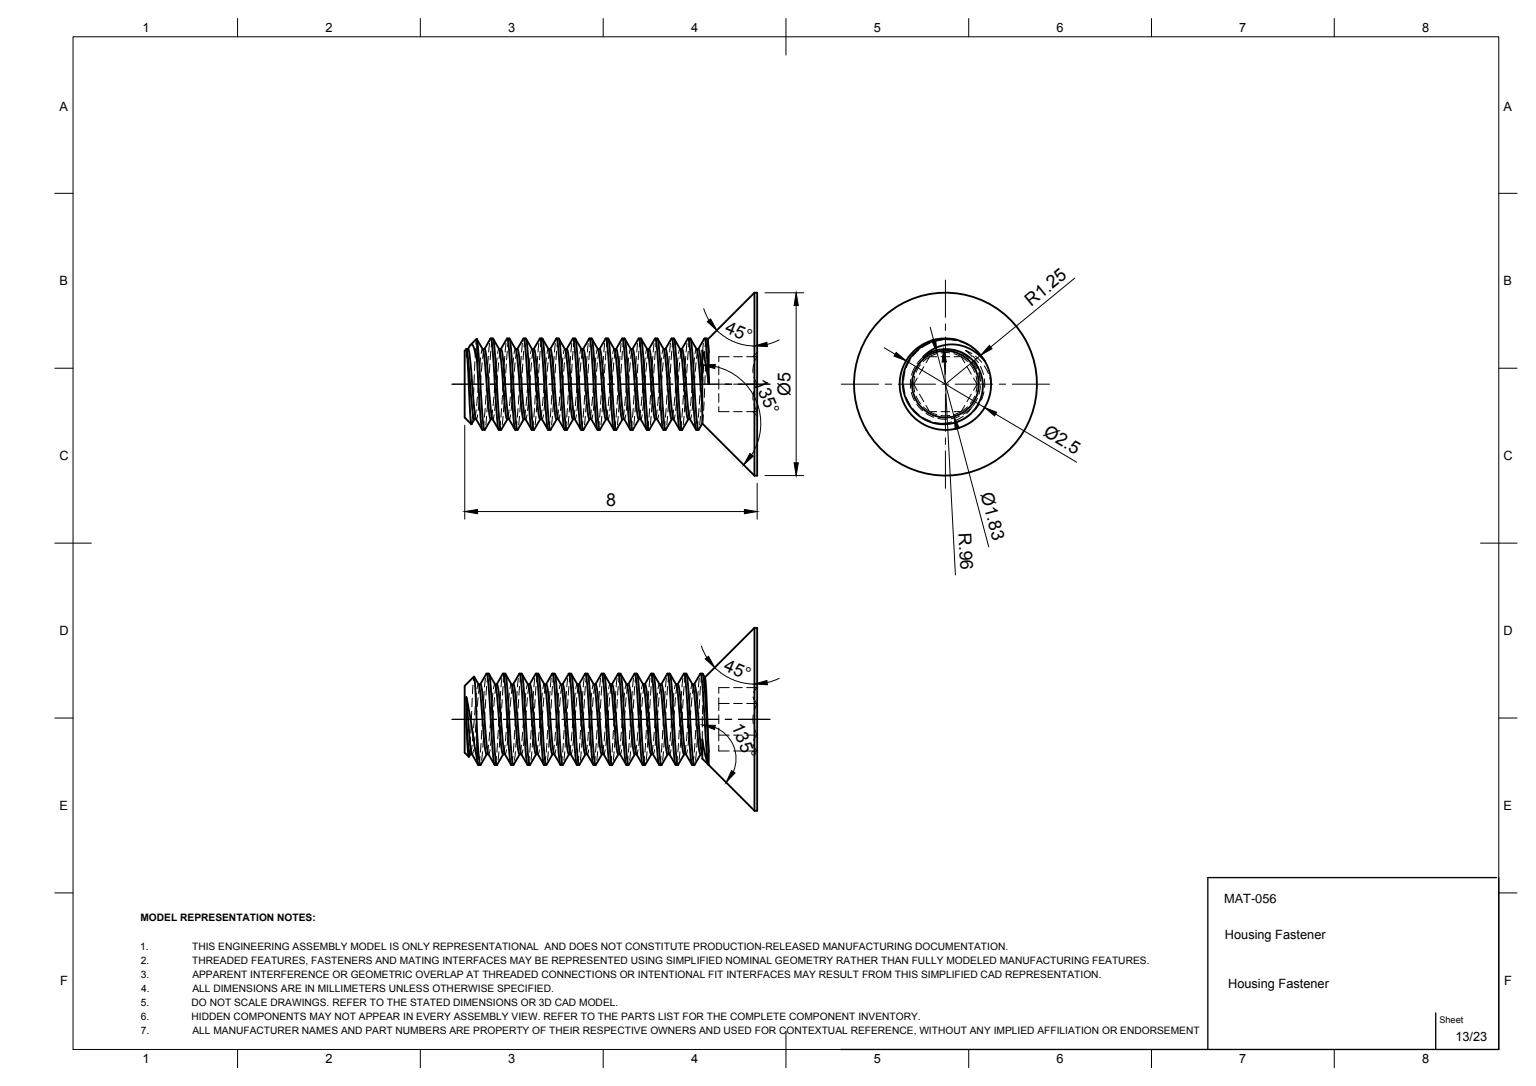
ISO-10303-21;
HEADER;
/* Generated by software containing ST-Developer
 * from STEP Tools, Inc. (www.steptools.com) 
 */

FILE_DESCRIPTION(
/* description */ (''),
/* implementation_level */ '2;1');

FILE_NAME(
/* name */ 'Housing Fastener.step',
/* time_stamp */ '2026-10-28T16:47:13+01:00',
/* author */ (''),
/* organization */ (''),
/* preprocessor_version */ 'ST-DEVELOPER v20.2',
/* originating_system */ 'Autodesk Translation Framework v15.17.0.0',
/* authorisation */ '');

FILE_SCHEMA (('AUTOMOTIVE_DESIGN { 1 0 10303 214 3 1 1 }'));
ENDSEC;

DATA;
#10=MECHANICAL_DESIGN_GEOMETRIC_PRESENTATION_REPRESENTATION('',(#4606),#459242);
#2317=(
BOUNDED_SURFACE()
B_SPLINE_SURFACE(1,2,((#370739,#370740,#370741,#370742,#370743,#370744,
#370745,#370746,#370747,#370748,#370749,#370750,#370751,#370752,#370753,
#370754,#370755,#370756,#370757,#370758,#370759,#370760,#370761,#370762,
#370763,#370764,#370765,#370766,#370767,#370768,#370769,#370770,#370771,
#370772,#370773,#370774,#370775,#370776,#370777,#370778,#370779,#370780,
#370781,#370782,#370783,#370784,#370785,#370786,#370787,#370788,#370789,
#370790,#370791,#370792,#370793,#370794,#370795,#370796,#370797,#370798,
#370799,#370800,#370801,#370802,#370803,#370804,#370805,#370806,#370807,
#370808,#370809,#370810,#370811,#370812,#370813,#370814,#370815,#370816,
#370817,#370818,#370819,#370820,#370821,#370822,#370823,#370824,#370825,
#370826,#370827,#370828,#370829,#370830,#370831,#370832,#370833,#370834,
#370835,#370836,#370837,#370838,#370839,#370840,#370841,#370842,#370843,
#370844,#370845,#370846,#370847,#370848,#370849,#370850,#370851,#370852,
#370853,#370854,#370855,#370856,#370857,#370858,#370859,#370860,#370861,
#370862,#370863,#370864,#370865,#370866,#370867,#370868,#370869,#370870,
#370871,#370872,#370873,#370874,#370875,#370876,#370877,#370878,#370879,
#370880,#370881,#370882,#370883,#370884,#370885,#370886,#370887,#370888,
#370889,#370890,#370891,#370892,#370893,#370894,#370895,#370896,#370897,
#370898,#370899,#370900,#370901,#370902,#370903,#370904,#370905,#370906,
#370907,#370908,#370909,#370910,#370911,#370912,#370913,#370914,#370915,
#370916,#370917,#370918,#370919,#370920,#370921,#370922,#370923,#370924,
#370925,#370926,#370927,#370928,#370929,#370930,#370931,#370932,#370933,
#370934,#370935,#370936,#370937,#370938,#370939,#370940,#370941,#370942,
#370943,#370944,#370945,#370946,#370947,#370948,#370949,#370950,#370951,
#370952,#370953,#370954,#370955),(#370956,#370957,#370958,#370959,#370960,
#370961,#370962,#370963,#370964,#370965,#370966,#370967,#370968,#370969,
#370970,#370971,#370972,#370973,#370974,#370975,#370976,#370977,#370978,
#370979,#370980,#370981,#370982,#370983,#370984,#370985,#370986,#370987,
#370988,#370989,#370990,#370991,#370992,#370993,#370994,#370995,#370996,
#370997,#370998,#370999,#371000,#371001,#371002,#371003,#371004,#371005,
#371006,#371007,#371008,#371009,#371010,#371011,#371012,#371013,#371014,
#371015,#371016,#371017,#371018,#371019,#371020,#371021,#371022,#371023,
#371024,#371025,#371026,#371027,#371028,#371029,#371030,#371031,#371032,
#371033,#371034,#371035,#371036,#371037,#371038,#371039,#371040,#371041,
#371042,#371043,#371044,#371045,#371046,#371047,#371048,#371049,#371050,
#371051,#371052,#371053,#371054,#371055,#371056,#371057,#371058,#371059,
#371060,#371061,#371062,#371063,#371064,#371065,#371066,#371067,#371068,
#371069,#371070,#371071,#371072,#371073,#371074,#371075,#371076,#371077,
#371078,#371079,#371080,#371081,#371082,#371083,#371084,#371085,#371086,
#371087,#371088,#371089,#371090,#371091,#371092,#371093,#371094,#371095,
#371096,#371097,#371098,#371099,#371100,#371101,#371102,#371103,#371104,
#371105,#371106,#371107,#371108,#371109,#371110,#371111,#371112,#371113,
#371114,#371115,#371116,#371117,#371118,#371119,#371120,#371121,#371122,
#371123,#371124,#371125,#371126,#371127,#371128,#371129,#371130,#371131,
#371132,#371133,#371134,#371135,#371136,#371137,#371138,#371139,#371140,
#371141,#371142,#371143,#371144,#371145,#371146,#371147,#371148,#371149,
#371150,#371151,#371152,#371153,#371154,#371155,#371156,#371157,#371158,
#371159,#371160,#371161,#371162,#371163,#371164,#371165,#371166,#371167,
#371168,#371169,#371170,#371171,#371172)),.UNSPECIFIED.,.F.,.F.,.F.)
B_SPLINE_SURFACE_WITH_KNOTS((2,2),(3,2,2,2,2,2,2,2,2,2,2,2,2,2,2,2,2,2,
2,2,2,2,2,2,2,2,2,2,2,2,2,2,2,2,2,2,2,2,2,2,2,2,2,2,2,2,2,2,2,2,2,2,2,2,
2,2,2,2,2,2,2,2,2,2,2,2,2,2,2,2,2,2,2,2,2,2,2,2,2,2,2,2,2,2,2,2,2,2,2,2,
2,2,2,2,2,2,2,2,2,2,2,2,2,2,2,2,2,2,3),(-1.08044907090275E-5,1.),(0.,0.00925925925925926,
0.0185185185185185,0.0277777777777778,0.037037037037037,0.0462962962962963,
0.0555555555555556,0.0648148148148148,0.0740740740740741,0.0833333333333333,
0.0925925925925926,0.101851851851852,0.111111111111111,0.12037037037037,
0.12962962962963,0.138888888888889,0.148148148148148,0.157407407407407,
0.166666666666667,0.175925925925926,0.185185185185185,0.194444444444444,
0.203703703703704,0.212962962962963,0.222222222222222,0.231481481481481,
0.240740740740741,0.25,0.259259259259259,0.268518518518519,0.277777777777778,
0.287037037037037,0.296296296296296,0.305555555555556,0.314814814814815,
0.324074074074074,0.333333333333333,0.342592592592593,0.351851851851852,
0.361111111111111,0.37037037037037,0.37962962962963,0.388888888888889,0.398148148148148,
0.407407407407407,0.416666666666667,0.425925925925926,0.435185185185185,
0.444444444444444,0.453703703703704,0.462962962962963,0.472222222222222,
0.481481481481481,0.490740740740741,0.5,0.509259259259259,0.518518518518518,
0.527777777777778,0.537037037037037,0.546296296296296,0.555555555555556,
0.564814814814815,0.574074074074074,0.583333333333333,0.592592592592593,
0.601851851851852,0.611111111111111,0.62037037037037,0.62962962962963,0.638888888888889,
0.648148148148148,0.657407407407407,0.666666666666667,0.675925925925926,
0.685185185185185,0.694444444444444,0.703703703703704,0.712962962962963,
0.722222222222222,0.731481481481482,0.740740740740741,0.75,0.759259259259259,
0.768518518518518,0.777777777777778,0.787037037037037,0.796296296296296,
0.805555555555556,0.814814814814815,0.824074074074074,0.833333333333333,
0.842592592592593,0.851851851851852,0.861111111111111,0.87037037037037,
0.87962962962963,0.888888888888889,0.898148148148148,0.907407407407407,
0.916666666666667,0.925925925925926,0.935185185185185,0.944444444444444,
0.953703703703704,0.962962962962963,0.972222222222222,0.981481481481482,
0.987622467374972,0.997498692048721),.UNSPECIFIED.)
GEOMETRIC_REPRESENTATION_ITEM()
RATIONAL_B_SPLINE_SURFACE(((1.,0.866025403784439,1.,0.866025403784439,1.,
0.866025403784439,1.,0.866025403784439,1.,0.866025403784439,1.,0.866025403784439,
1.,0.866025403784439,1.,0.866025403784439,1.,0.866025403784439,1.,0.866025403784439,
1.,0.866025403784439,1.,0.866025403784439,1.,0.866025403784439,1.,0.866025403784439,
1.,0.866025403784439,1.,0.866025403784439,1.,0.866025403784439,1.,0.866025403784439,
1.,0.866025403784439,1.,0.866025403784439,1.,0.866025403784439,1.,0.866025403784439,
1.,0.866025403784439,1.,0.866025403784439,1.,0.866025403784439,1.,0.866025403784439,
1.,0.866025403784439,1.,0.866025403784439,1.,0.866025403784439,1.,0.866025403784439,
1.,0.866025403784439,1.,0.866025403784439,1.,0.866025403784439,1.,0.866025403784439,
1.,0.866025403784439,1.,0.866025403784439,1.,0.866025403784439,1.,0.866025403784439,
1.,0.866025403784439,1.,0.866025403784439,1.,0.866025403784439,1.,0.866025403784439,
1.,0.866025403784439,1.,0.866025403784439,1.,0.866025403784439,1.,0.866025403784439,
1.,0.866025403784439,1.,0.866025403784439,1.,0.866025403784439,1.,0.866025403784439,
1.,0.866025403784439,1.,0.866025403784439,1.,0.866025403784439,1.,0.866025403784439,
1.,0.866025403784439,1.,0.866025403784439,1.,0.866025403784439,1.,0.866025403784439,
1.,0.866025403784439,1.,0.866025403784439,1.,0.866025403784439,1.,0.866025403784439,
1.,0.866025403784439,1.,0.866025403784439,1.,0.866025403784439,1.,0.866025403784439,
1.,0.866025403784439,1.,0.866025403784439,1.,0.866025403784439,1.,0.866025403784439,
1.,0.866025403784439,1.,0.866025403784439,1.,0.866025403784439,1.,0.866025403784439,
1.,0.866025403784439,1.,0.866025403784439,1.,0.866025403784439,1.,0.866025403784439,
1.,0.866025403784439,1.,0.866025403784439,1.,0.866025403784439,1.,0.866025403784439,
1.,0.866025403784439,1.,0.866025403784439,1.,0.866025403784439,1.,0.866025403784439,
1.,0.866025403784439,1.,0.866025403784439,1.,0.866025403784439,1.,0.866025403784439,
1.,0.866025403784439,1.,0.866025403784439,1.,0.866025403784439,1.,0.866025403784439,
1.,0.866025403784439,1.,0.866025403784439,1.,0.866025403784439,1.,0.866025403784439,
1.,0.866025403784439,1.,0.866025403784439,1.,0.866025403784439,1.,0.866025403784439,
1.,0.866025403784439,1.,0.866025403784439,1.,0.866025403784439,1.,0.866025403784439,
1.,0.911144500611853,0.940151640776859,0.940151640776859,0.940151640776859),
(1.,0.866025403784439,1.,0.866025403784439,1.,0.866025403784439,1.,0.866025403784439,
1.,0.866025403784439,1.,0.866025403784439,1.,0.866025403784439,1.,0.866025403784439,
1.,0.866025403784439,1.,0.866025403784439,1.,0.866025403784439,1.,0.866025403784439,
1.,0.866025403784439,1.,0.866025403784439,1.,0.866025403784439,1.,0.866025403784439,
1.,0.866025403784439,1.,0.866025403784439,1.,0.866025403784439,1.,0.866025403784439,
1.,0.866025403784439,1.,0.866025403784439,1.,0.866025403784439,1.,0.866025403784439,
1.,0.866025403784439,1.,0.866025403784439,1.,0.866025403784439,1.,0.866025403784439,
1.,0.866025403784439,1.,0.866025403784439,1.,0.866025403784439,1.,0.866025403784439,
1.,0.866025403784439,1.,0.866025403784439,1.,0.866025403784439,1.,0.866025403784439,
1.,0.866025403784439,1.,0.866025403784439,1.,0.866025403784439,1.,0.866025403784439,
1.,0.866025403784439,1.,0.866025403784439,1.,0.866025403784439,1.,0.866025403784439,
1.,0.866025403784439,1.,0.866025403784439,1.,0.866025403784439,1.,0.866025403784439,
1.,0.866025403784439,1.,0.866025403784439,1.,0.866025403784439,1.,0.866025403784439,
1.,0.866025403784439,1.,0.866025403784439,1.,0.866025403784439,1.,0.866025403784439,
1.,0.866025403784439,1.,0.866025403784439,1.,0.866025403784439,1.,0.866025403784439,
1.,0.866025403784439,1.,0.866025403784439,1.,0.866025403784439,1.,0.866025403784439,
1.,0.866025403784439,1.,0.866025403784439,1.,0.866025403784439,1.,0.866025403784439,
1.,0.866025403784439,1.,0.866025403784439,1.,0.866025403784439,1.,0.866025403784439,
1.,0.866025403784439,1.,0.866025403784439,1.,0.866025403784439,1.,0.866025403784439,
1.,0.866025403784439,1.,0.866025403784439,1.,0.866025403784439,1.,0.866025403784439,
1.,0.866025403784439,1.,0.866025403784439,1.,0.866025403784439,1.,0.866025403784439,
1.,0.866025403784439,1.,0.866025403784439,1.,0.866025403784439,1.,0.866025403784439,
1.,0.866025403784439,1.,0.866025403784439,1.,0.866025403784439,1.,0.866025403784439,
1.,0.866025403784439,1.,0.866025403784439,1.,0.866025403784439,1.,0.866025403784439,
1.,0.866025403784439,1.,0.866025403784439,1.,0.866025403784439,1.,0.866025403784439,
1.,0.866025403784439,1.,0.866025403784439,1.,0.866025403784439,1.,0.866025403784439,
1.,0.866025403784439,1.,0.866025403784439,1.,0.911144500611853,0.940151640776859,
0.940151640776859,0.940151640776859)))
REPRESENTATION_ITEM('')
SURFACE()
);
#2318=(
BOUNDED_SURFACE()
B_SPLINE_SURFACE(1,2,((#371177,#371178,#371179,#371180,#371181,#371182,
#371183,#371184,#371185,#371186,#371187,#371188,#371189,#371190,#371191,
#371192,#371193,#371194,#371195,#371196,#371197,#371198,#371199,#371200,
#371201,#371202,#371203,#371204,#371205,#371206,#371207,#371208,#371209,
#371210,#371211,#371212,#371213,#371214,#371215,#371216,#371217,#371218,
#371219,#371220,#371221,#371222,#371223,#371224,#371225,#371226,#371227,
#371228,#371229,#371230,#371231,#371232,#371233,#371234,#371235,#371236,
#371237,#371238,#371239,#371240,#371241,#371242,#371243,#371244,#371245,
#371246,#371247,#371248,#371249,#371250,#371251,#371252,#371253,#371254,
#371255,#371256,#371257,#371258,#371259,#371260,#371261,#371262,#371263,
#371264,#371265,#371266,#371267,#371268,#371269,#371270,#371271,#371272,
#371273,#371274,#371275,#371276,#371277,#371278,#371279,#371280,#371281,
#371282,#371283,#371284,#371285,#371286,#371287,#371288,#371289,#371290,
#371291,#371292,#371293,#371294,#371295,#371296,#371297,#371298,#371299,
#371300,#371301,#371302,#371303,#371304,#371305,#371306,#371307,#371308,
#371309,#371310,#371311,#371312,#371313,#371314,#371315,#371316,#371317,
#371318,#371319,#371320,#371321,#371322,#371323,#371324,#371325,#371326,
#371327,#371328,#371329,#371330,#371331,#371332,#371333,#371334,#371335,
#371336,#371337,#371338,#371339,#371340,#371341,#371342,#371343,#371344,
#371345,#371346,#371347,#371348,#371349,#371350,#371351,#371352,#371353,
#371354,#371355,#371356,#371357,#371358,#371359,#371360,#371361,#371362,
#371363,#371364,#371365,#371366,#371367,#371368,#371369,#371370,#371371,
#371372,#371373,#371374,#371375,#371376,#371377,#371378,#371379,#371380,
#371381,#371382,#371383,#371384,#371385,#371386,#371387,#371388,#371389,
#371390,#371391),(#371392,#371393,#371394,#371395,#371396,#371397,#371398,
#371399,#371400,#371401,#371402,#371403,#371404,#371405,#371406,#371407,
#371408,#371409,#371410,#371411,#371412,#371413,#371414,#371415,#371416,
#371417,#371418,#371419,#371420,#371421,#371422,#371423,#371424,#371425,
#371426,#371427,#371428,#371429,#371430,#371431,#371432,#371433,#371434,
#371435,#371436,#371437,#371438,#371439,#371440,#371441,#371442,#371443,
#371444,#371445,#371446,#371447,#371448,#371449,#371450,#371451,#371452,
#371453,#371454,#371455,#371456,#371457,#371458,#371459,#371460,#371461,
#371462,#371463,#371464,#371465,#371466,#371467,#371468,#371469,#371470,
#371471,#371472,#371473,#371474,#371475,#371476,#371477,#371478,#371479,
#371480,#371481,#371482,#371483,#371484,#371485,#371486,#371487,#371488,
#371489,#371490,#371491,#371492,#371493,#371494,#371495,#371496,#371497,
#371498,#371499,#371500,#371501,#371502,#371503,#371504,#371505,#371506,
#371507,#371508,#371509,#371510,#371511,#371512,#371513,#371514,#371515,
#371516,#371517,#371518,#371519,#371520,#371521,#371522,#371523,#371524,
#371525,#371526,#371527,#371528,#371529,#371530,#371531,#371532,#371533,
#371534,#371535,#371536,#371537,#371538,#371539,#371540,#371541,#371542,
#371543,#371544,#371545,#371546,#371547,#371548,#371549,#371550,#371551,
#371552,#371553,#371554,#371555,#371556,#371557,#371558,#371559,#371560,
#371561,#371562,#371563,#371564,#371565,#371566,#371567,#371568,#371569,
#371570,#371571,#371572,#371573,#371574,#371575,#371576,#371577,#371578,
#371579,#371580,#371581,#371582,#371583,#371584,#371585,#371586,#371587,
#371588,#371589,#371590,#371591,#371592,#371593,#371594,#371595,#371596,
#371597,#371598,#371599,#371600,#371601,#371602,#371603,#371604,#371605,
#371606)),.UNSPECIFIED.,.F.,.F.,.F.)
B_SPLINE_SURFACE_WITH_KNOTS((2,2),(3,2,2,2,2,2,2,2,2,2,2,2,2,2,2,2,2,2,
2,2,2,2,2,2,2,2,2,2,2,2,2,2,2,2,2,2,2,2,2,2,2,2,2,2,2,2,2,2,2,2,2,2,2,2,
2,2,2,2,2,2,2,2,2,2,2,2,2,2,2,2,2,2,2,2,2,2,2,2,2,2,2,2,2,2,2,2,2,2,2,2,
2,2,2,2,2,2,2,2,2,2,2,2,2,2,2,2,2,3),(0.,1.),(0.,0.00925925925925926,0.0185185185185185,
0.0277777777777778,0.037037037037037,0.0462962962962963,0.0555555555555556,
0.0648148148148148,0.0740740740740741,0.0833333333333333,0.0925925925925926,
0.101851851851852,0.111111111111111,0.12037037037037,0.12962962962963,0.138888888888889,
0.148148148148148,0.157407407407407,0.166666666666667,0.175925925925926,
0.185185185185185,0.194444444444444,0.203703703703704,0.212962962962963,
0.222222222222222,0.231481481481481,0.240740740740741,0.25,0.259259259259259,
0.268518518518519,0.277777777777778,0.287037037037037,0.296296296296296,
0.305555555555556,0.314814814814815,0.324074074074074,0.333333333333333,
0.342592592592593,0.351851851851852,0.361111111111111,0.37037037037037,
0.37962962962963,0.388888888888889,0.398148148148148,0.407407407407407,
0.416666666666667,0.425925925925926,0.435185185185185,0.444444444444444,
0.453703703703704,0.462962962962963,0.472222222222222,0.481481481481481,
0.490740740740741,0.5,0.509259259259259,0.518518518518518,0.527777777777778,
0.537037037037037,0.546296296296296,0.555555555555556,0.564814814814815,
0.574074074074074,0.583333333333333,0.592592592592593,0.601851851851852,
0.611111111111111,0.62037037037037,0.62962962962963,0.638888888888889,0.648148148148148,
0.657407407407407,0.666666666666667,0.675925925925926,0.685185185185185,
0.694444444444444,0.703703703703704,0.712962962962963,0.722222222222222,
0.731481481481482,0.740740740740741,0.75,0.759259259259259,0.768518518518518,
0.777777777777778,0.787037037037037,0.796296296296296,0.805555555555556,
0.814814814814815,0.824074074074074,0.833333333333333,0.842592592592593,
0.851851851851852,0.861111111111111,0.87037037037037,0.87962962962963,0.888888888888889,
0.898148148148148,0.907407407407407,0.916666666666667,0.925925925925926,
0.935185185185185,0.944444444444444,0.953703703703704,0.962962962962963,
0.972222222222222,0.981481481481482,0.987622586258463),.UNSPECIFIED.)
GEOMETRIC_REPRESENTATION_ITEM()
RATIONAL_B_SPLINE_SURFACE(((1.,0.866025403784439,1.,0.866025403784439,1.,
0.866025403784439,1.,0.866025403784439,1.,0.866025403784439,1.,0.866025403784439,
1.,0.866025403784439,1.,0.866025403784439,1.,0.866025403784439,1.,0.866025403784439,
1.,0.866025403784439,1.,0.866025403784439,1.,0.866025403784439,1.,0.866025403784439,
1.,0.866025403784439,1.,0.866025403784439,1.,0.866025403784439,1.,0.866025403784439,
1.,0.866025403784439,1.,0.866025403784439,1.,0.866025403784439,1.,0.866025403784439,
1.,0.866025403784439,1.,0.866025403784439,1.,0.866025403784439,1.,0.866025403784439,
1.,0.866025403784439,1.,0.866025403784439,1.,0.866025403784439,1.,0.866025403784439,
1.,0.866025403784439,1.,0.866025403784439,1.,0.866025403784439,1.,0.866025403784439,
1.,0.866025403784439,1.,0.866025403784439,1.,0.866025403784439,1.,0.866025403784439,
1.,0.866025403784439,1.,0.866025403784439,1.,0.866025403784439,1.,0.866025403784439,
1.,0.866025403784439,1.,0.866025403784439,1.,0.866025403784439,1.,0.866025403784439,
1.,0.866025403784439,1.,0.866025403784439,1.,0.866025403784439,1.,0.866025403784439,
1.,0.866025403784439,1.,0.866025403784439,1.,0.866025403784439,1.,0.866025403784439,
1.,0.866025403784439,1.,0.866025403784439,1.,0.866025403784439,1.,0.866025403784439,
1.,0.866025403784439,1.,0.866025403784439,1.,0.866025403784439,1.,0.866025403784439,
1.,0.866025403784439,1.,0.866025403784439,1.,0.866025403784439,1.,0.866025403784439,
1.,0.866025403784439,1.,0.866025403784439,1.,0.866025403784439,1.,0.866025403784439,
1.,0.866025403784439,1.,0.866025403784439,1.,0.866025403784439,1.,0.866025403784439,
1.,0.866025403784439,1.,0.866025403784439,1.,0.866025403784439,1.,0.866025403784439,
1.,0.866025403784439,1.,0.866025403784439,1.,0.866025403784439,1.,0.866025403784439,
1.,0.866025403784439,1.,0.866025403784439,1.,0.866025403784439,1.,0.866025403784439,
1.,0.866025403784439,1.,0.866025403784439,1.,0.866025403784439,1.,0.866025403784439,
1.,0.866025403784439,1.,0.866025403784439,1.,0.866025403784439,1.,0.866025403784439,
1.,0.866025403784439,1.,0.866025403784439,1.,0.866025403784439,1.,0.866025403784439,
1.,0.866025403784439,1.,0.866025403784439,1.,0.866025403784439,1.,0.866025403784439,
1.,0.866025403784439,1.,0.866025403784439,1.,0.866025403784439,1.,0.866025403784439,
1.,0.911142780456138,0.940152763920857),(1.,0.866025403784439,1.,0.866025403784439,
1.,0.866025403784439,1.,0.866025403784439,1.,0.866025403784439,1.,0.866025403784439,
1.,0.866025403784439,1.,0.866025403784439,1.,0.866025403784439,1.,0.866025403784439,
1.,0.866025403784439,1.,0.866025403784439,1.,0.866025403784439,1.,0.866025403784439,
1.,0.866025403784439,1.,0.866025403784439,1.,0.866025403784439,1.,0.866025403784439,
1.,0.866025403784439,1.,0.866025403784439,1.,0.866025403784439,1.,0.866025403784439,
1.,0.866025403784439,1.,0.866025403784439,1.,0.866025403784439,1.,0.866025403784439,
1.,0.866025403784439,1.,0.866025403784439,1.,0.866025403784439,1.,0.866025403784439,
1.,0.866025403784439,1.,0.866025403784439,1.,0.866025403784439,1.,0.866025403784439,
1.,0.866025403784439,1.,0.866025403784439,1.,0.866025403784439,1.,0.866025403784439,
1.,0.866025403784439,1.,0.866025403784439,1.,0.866025403784439,1.,0.866025403784439,
1.,0.866025403784439,1.,0.866025403784439,1.,0.866025403784439,1.,0.866025403784439,
1.,0.866025403784439,1.,0.866025403784439,1.,0.866025403784439,1.,0.866025403784439,
1.,0.866025403784439,1.,0.866025403784439,1.,0.866025403784439,1.,0.866025403784439,
1.,0.866025403784439,1.,0.866025403784439,1.,0.866025403784439,1.,0.866025403784439,
1.,0.866025403784439,1.,0.866025403784439,1.,0.866025403784439,1.,0.866025403784439,
1.,0.866025403784439,1.,0.866025403784439,1.,0.866025403784439,1.,0.866025403784439,
1.,0.866025403784439,1.,0.866025403784439,1.,0.866025403784439,1.,0.866025403784439,
1.,0.866025403784439,1.,0.866025403784439,1.,0.866025403784439,1.,0.866025403784439,
1.,0.866025403784439,1.,0.866025403784439,1.,0.866025403784439,1.,0.866025403784439,
1.,0.866025403784439,1.,0.866025403784439,1.,0.866025403784439,1.,0.866025403784439,
1.,0.866025403784439,1.,0.866025403784439,1.,0.866025403784439,1.,0.866025403784439,
1.,0.866025403784439,1.,0.866025403784439,1.,0.866025403784439,1.,0.866025403784439,
1.,0.866025403784439,1.,0.866025403784439,1.,0.866025403784439,1.,0.866025403784439,
1.,0.866025403784439,1.,0.866025403784439,1.,0.866025403784439,1.,0.866025403784439,
1.,0.866025403784439,1.,0.866025403784439,1.,0.866025403784439,1.,0.866025403784439,
1.,0.866025403784439,1.,0.866025403784439,1.,0.866025403784439,1.,0.866025403784439,
1.,0.911142780456138,0.940152763920857)))
REPRESENTATION_ITEM('')
SURFACE()
);
#4224=(
BOUNDED_CURVE()
B_SPLINE_CURVE(2,(#368993,#368994,#368995,#368996,#368997,#368998,#368999),
 .UNSPECIFIED.,.F.,.F.)
B_SPLINE_CURVE_WITH_KNOTS((3,2,2,3),(0.815651079918082,0.825026379687255,
0.834401679456429,0.840557475565081),.UNSPECIFIED.)
CURVE()
GEOMETRIC_REPRESENTATION_ITEM()
RATIONAL_B_SPLINE_CURVE((1.,0.866025403784439,1.,0.866025403784439,1.,0.912032647664899,
0.939583539764693))
REPRESENTATION_ITEM('')
);
#4225=(
BOUNDED_CURVE()
B_SPLINE_CURVE(2,(#369002,#369003,#369004,#369005,#369006),
 .UNSPECIFIED.,.F.,.F.)
B_SPLINE_CURVE_WITH_KNOTS((3,2,3),(0.815651208026079,0.825026509267758,
0.833532478045858),.UNSPECIFIED.)
CURVE()
GEOMETRIC_REPRESENTATION_ITEM()
RATIONAL_B_SPLINE_CURVE((1.,0.866025403784439,1.,0.878448307623234,0.977458040128596))
REPRESENTATION_ITEM('')
);
#4226=(
BOUNDED_CURVE()
B_SPLINE_CURVE(2,(#369011,#369012,#369013,#369014,#369015,#369016,#369017,
#369018,#369019,#369020,#369021,#369022,#369023),.UNSPECIFIED.,.F.,.F.)
B_SPLINE_CURVE_WITH_KNOTS((3,2,2,2,2,2,3),(0.759399281303043,0.768774581072216,
0.778149880841389,0.787525180610563,0.796900480379736,0.806275780148909,
0.815651079918082),.UNSPECIFIED.)
CURVE()
GEOMETRIC_REPRESENTATION_ITEM()
RATIONAL_B_SPLINE_CURVE((1.,0.866025403784439,1.,0.866025403784439,1.,0.866025403784439,
1.,0.866025403784439,1.,0.866025403784439,1.,0.866025403784439,1.))
REPRESENTATION_ITEM('')
);
#4227=(
BOUNDED_CURVE()
B_SPLINE_CURVE(2,(#369024,#369025,#369026,#369027,#369028,#369029,#369030,
#369031,#369032,#369033,#369034,#369035,#369036),.UNSPECIFIED.,.F.,.F.)
B_SPLINE_CURVE_WITH_KNOTS((3,2,2,2,2,2,3),(0.759399400576005,0.768774701817684,
0.778150003059363,0.787525304301042,0.796900605542721,0.8062759067844,0.815651208026079),
 .UNSPECIFIED.)
CURVE()
GEOMETRIC_REPRESENTATION_ITEM()
RATIONAL_B_SPLINE_CURVE((1.,0.866025403784439,1.,0.866025403784439,1.,0.866025403784439,
1.,0.866025403784439,1.,0.866025403784439,1.,0.866025403784439,1.))
REPRESENTATION_ITEM('')
);
#4228=(
BOUNDED_CURVE()
B_SPLINE_CURVE(2,(#369041,#369042,#369043,#369044,#369045,#369046,#369047,
#369048,#369049,#369050,#369051,#369052,#369053),.UNSPECIFIED.,.F.,.F.)
B_SPLINE_CURVE_WITH_KNOTS((3,2,2,2,2,2,3),(0.703147482688004,0.712522782457177,
0.72189808222635,0.731273381995523,0.740648681764697,0.75002398153387,0.759399281303043),
 .UNSPECIFIED.)
CURVE()
GEOMETRIC_REPRESENTATION_ITEM()
RATIONAL_B_SPLINE_CURVE((1.,0.866025403784439,1.,0.866025403784439,1.,0.866025403784439,
1.,0.866025403784439,1.,0.866025403784439,1.,0.866025403784439,1.))
REPRESENTATION_ITEM('')
);
#4229=(
BOUNDED_CURVE()
B_SPLINE_CURVE(2,(#369054,#369055,#369056,#369057,#369058,#369059,#369060,
#369061,#369062,#369063,#369064,#369065,#369066),.UNSPECIFIED.,.F.,.F.)
B_SPLINE_CURVE_WITH_KNOTS((3,2,2,2,2,2,3),(0.70314759312593,0.712522894367609,
0.721898195609288,0.731273496850967,0.740648798092646,0.750024099334325,
0.759399400576005),.UNSPECIFIED.)
CURVE()
GEOMETRIC_REPRESENTATION_ITEM()
RATIONAL_B_SPLINE_CURVE((1.,0.866025403784439,1.,0.866025403784439,1.,0.866025403784439,
1.,0.866025403784439,1.,0.866025403784439,1.,0.866025403784439,1.))
REPRESENTATION_ITEM('')
);
#4230=(
BOUNDED_CURVE()
B_SPLINE_CURVE(2,(#369071,#369072,#369073,#369074,#369075,#369076,#369077,
#369078,#369079,#369080,#369081,#369082,#369083),.UNSPECIFIED.,.F.,.F.)
B_SPLINE_CURVE_WITH_KNOTS((3,2,2,2,2,2,3),(0.646895684072964,0.656270983842138,
0.665646283611311,0.675021583380484,0.684396883149657,0.693772182918831,
0.703147482688004),.UNSPECIFIED.)
CURVE()
GEOMETRIC_REPRESENTATION_ITEM()
RATIONAL_B_SPLINE_CURVE((1.,0.866025403784439,1.,0.866025403784439,1.,0.866025403784439,
1.,0.866025403784439,1.,0.866025403784439,1.,0.866025403784439,1.))
REPRESENTATION_ITEM('')
);
#4231=(
BOUNDED_CURVE()
B_SPLINE_CURVE(2,(#369084,#369085,#369086,#369087,#369088,#369089,#369090,
#369091,#369092,#369093,#369094,#369095,#369096),.UNSPECIFIED.,.F.,.F.)
B_SPLINE_CURVE_WITH_KNOTS((3,2,2,2,2,2,3),(0.646895785675856,0.656271086917535,
0.665646388159214,0.675021689400893,0.684396990642572,0.693772291884251,
0.70314759312593),.UNSPECIFIED.)
CURVE()
GEOMETRIC_REPRESENTATION_ITEM()
RATIONAL_B_SPLINE_CURVE((1.,0.866025403784439,1.,0.866025403784439,1.,0.866025403784439,
1.,0.866025403784439,1.,0.866025403784439,1.,0.866025403784439,1.))
REPRESENTATION_ITEM('')
);
#4232=(
BOUNDED_CURVE()
B_SPLINE_CURVE(2,(#369101,#369102,#369103,#369104,#369105,#369106,#369107,
#369108,#369109,#369110,#369111,#369112,#369113),.UNSPECIFIED.,.F.,.F.)
B_SPLINE_CURVE_WITH_KNOTS((3,2,2,2,2,2,3),(0.590643885457925,0.600019185227099,
0.609394484996272,0.618769784765445,0.628145084534618,0.637520384303791,
0.646895684072964),.UNSPECIFIED.)
CURVE()
GEOMETRIC_REPRESENTATION_ITEM()
RATIONAL_B_SPLINE_CURVE((1.,0.866025403784439,1.,0.866025403784439,1.,0.866025403784439,
1.,0.866025403784439,1.,0.866025403784439,1.,0.866025403784439,1.))
REPRESENTATION_ITEM('')
);
#4233=(
BOUNDED_CURVE()
B_SPLINE_CURVE(2,(#369114,#369115,#369116,#369117,#369118,#369119,#369120,
#369121,#369122,#369123,#369124,#369125,#369126),.UNSPECIFIED.,.F.,.F.)
B_SPLINE_CURVE_WITH_KNOTS((3,2,2,2,2,2,3),(0.590643978225781,0.60001927946746,
0.60939458070914,0.618769881950819,0.628145183192497,0.637520484434177,
0.646895785675856),.UNSPECIFIED.)
CURVE()
GEOMETRIC_REPRESENTATION_ITEM()
RATIONAL_B_SPLINE_CURVE((1.,0.866025403784439,1.,0.866025403784439,1.,0.866025403784439,
1.,0.866025403784439,1.,0.866025403784439,1.,0.866025403784439,1.))
REPRESENTATION_ITEM('')
);
#4234=(
BOUNDED_CURVE()
B_SPLINE_CURVE(2,(#369131,#369132,#369133,#369134,#369135,#369136,#369137,
#369138,#369139,#369140,#369141,#369142,#369143),.UNSPECIFIED.,.F.,.F.)
B_SPLINE_CURVE_WITH_KNOTS((3,2,2,2,2,2,3),(0.534392086842886,0.543767386612059,
0.553142686381232,0.562517986150406,0.571893285919579,0.581268585688752,
0.590643885457925),.UNSPECIFIED.)
CURVE()
GEOMETRIC_REPRESENTATION_ITEM()
RATIONAL_B_SPLINE_CURVE((1.,0.866025403784439,1.,0.866025403784439,1.,0.866025403784439,
1.,0.866025403784439,1.,0.866025403784439,1.,0.866025403784439,1.))
REPRESENTATION_ITEM('')
);
#4235=(
BOUNDED_CURVE()
B_SPLINE_CURVE(2,(#369144,#369145,#369146,#369147,#369148,#369149,#369150,
#369151,#369152,#369153,#369154,#369155,#369156),.UNSPECIFIED.,.F.,.F.)
B_SPLINE_CURVE_WITH_KNOTS((3,2,2,2,2,2,3),(0.534392170775707,0.543767472017386,
0.553142773259065,0.562518074500744,0.571893375742423,0.581268676984102,
0.590643978225781),.UNSPECIFIED.)
CURVE()
GEOMETRIC_REPRESENTATION_ITEM()
RATIONAL_B_SPLINE_CURVE((1.,0.866025403784439,1.,0.866025403784439,1.,0.866025403784439,
1.,0.866025403784439,1.,0.866025403784439,1.,0.866025403784439,1.))
REPRESENTATION_ITEM('')
);
#4236=(
BOUNDED_CURVE()
B_SPLINE_CURVE(2,(#369161,#369162,#369163,#369164,#369165,#369166,#369167,
#369168,#369169,#369170,#369171,#369172,#369173),.UNSPECIFIED.,.F.,.F.)
B_SPLINE_CURVE_WITH_KNOTS((3,2,2,2,2,2,3),(0.478140288227847,0.48751558799702,
0.496890887766193,0.506266187535366,0.51564148730454,0.525016787073713,
0.534392086842886),.UNSPECIFIED.)
CURVE()
GEOMETRIC_REPRESENTATION_ITEM()
RATIONAL_B_SPLINE_CURVE((1.,0.866025403784439,1.,0.866025403784439,1.,0.866025403784439,
1.,0.866025403784439,1.,0.866025403784439,1.,0.866025403784439,1.))
REPRESENTATION_ITEM('')
);
#4237=(
BOUNDED_CURVE()
B_SPLINE_CURVE(2,(#369174,#369175,#369176,#369177,#369178,#369179,#369180,
#369181,#369182,#369183,#369184,#369185,#369186),.UNSPECIFIED.,.F.,.F.)
B_SPLINE_CURVE_WITH_KNOTS((3,2,2,2,2,2,3),(0.478140363325633,0.487515664567311,
0.496890965808991,0.50626626705067,0.515641568292349,0.525016869534028,
0.534392170775707),.UNSPECIFIED.)
CURVE()
GEOMETRIC_REPRESENTATION_ITEM()
RATIONAL_B_SPLINE_CURVE((1.,0.866025403784439,1.,0.866025403784439,1.,0.866025403784439,
1.,0.866025403784439,1.,0.866025403784439,1.,0.866025403784439,1.))
REPRESENTATION_ITEM('')
);
#4238=(
BOUNDED_CURVE()
B_SPLINE_CURVE(2,(#369191,#369192,#369193,#369194,#369195,#369196,#369197,
#369198,#369199,#369200,#369201,#369202,#369203),.UNSPECIFIED.,.F.,.F.)
B_SPLINE_CURVE_WITH_KNOTS((3,2,2,2,2,2,3),(0.421888489612808,0.431263789381981,
0.440639089151154,0.450014388920327,0.4593896886895,0.468764988458674,0.478140288227847),
 .UNSPECIFIED.)
CURVE()
GEOMETRIC_REPRESENTATION_ITEM()
RATIONAL_B_SPLINE_CURVE((1.,0.866025403784439,1.,0.866025403784439,1.,0.866025403784439,
1.,0.866025403784439,1.,0.866025403784439,1.,0.866025403784439,1.))
REPRESENTATION_ITEM('')
);
#4239=(
BOUNDED_CURVE()
B_SPLINE_CURVE(2,(#369204,#369205,#369206,#369207,#369208,#369209,#369210,
#369211,#369212,#369213,#369214,#369215,#369216),.UNSPECIFIED.,.F.,.F.)
B_SPLINE_CURVE_WITH_KNOTS((3,2,2,2,2,2,3),(0.421888555875558,0.431263857117237,
0.440639158358916,0.450014459600595,0.459389760842274,0.468765062083953,
0.478140363325633),.UNSPECIFIED.)
CURVE()
GEOMETRIC_REPRESENTATION_ITEM()
RATIONAL_B_SPLINE_CURVE((1.,0.866025403784439,1.,0.866025403784439,1.,0.866025403784439,
1.,0.866025403784439,1.,0.866025403784439,1.,0.866025403784439,1.))
REPRESENTATION_ITEM('')
);
#4240=(
BOUNDED_CURVE()
B_SPLINE_CURVE(2,(#369221,#369222,#369223,#369224,#369225,#369226,#369227,
#369228,#369229,#369230,#369231,#369232,#369233),.UNSPECIFIED.,.F.,.F.)
B_SPLINE_CURVE_WITH_KNOTS((3,2,2,2,2,2,3),(0.365636690997768,0.375011990766941,
0.384387290536115,0.393762590305288,0.403137890074461,0.412513189843634,
0.421888489612808),.UNSPECIFIED.)
CURVE()
GEOMETRIC_REPRESENTATION_ITEM()
RATIONAL_B_SPLINE_CURVE((1.,0.866025403784439,1.,0.866025403784439,1.,0.866025403784439,
1.,0.866025403784439,1.,0.866025403784439,1.,0.866025403784439,1.))
REPRESENTATION_ITEM('')
);
#4241=(
BOUNDED_CURVE()
B_SPLINE_CURVE(2,(#369234,#369235,#369236,#369237,#369238,#369239,#369240,
#369241,#369242,#369243,#369244,#369245,#369246),.UNSPECIFIED.,.F.,.F.)
B_SPLINE_CURVE_WITH_KNOTS((3,2,2,2,2,2,3),(0.365636748425484,0.375012049667163,
0.384387350908842,0.393762652150521,0.4031379533922,0.412513254633879,0.421888555875558),
 .UNSPECIFIED.)
CURVE()
GEOMETRIC_REPRESENTATION_ITEM()
RATIONAL_B_SPLINE_CURVE((1.,0.866025403784439,1.,0.866025403784439,1.,0.866025403784439,
1.,0.866025403784439,1.,0.866025403784439,1.,0.866025403784439,1.))
REPRESENTATION_ITEM('')
);
#4242=(
BOUNDED_CURVE()
B_SPLINE_CURVE(2,(#369251,#369252,#369253,#369254,#369255,#369256,#369257,
#369258,#369259,#369260,#369261,#369262,#369263),.UNSPECIFIED.,.F.,.F.)
B_SPLINE_CURVE_WITH_KNOTS((3,2,2,2,2,2,3),(0.309384892382729,0.318760192151902,
0.328135491921075,0.337510791690249,0.346886091459422,0.356261391228595,
0.365636690997768),.UNSPECIFIED.)
CURVE()
GEOMETRIC_REPRESENTATION_ITEM()
RATIONAL_B_SPLINE_CURVE((1.,0.866025403784439,1.,0.866025403784439,1.,0.866025403784439,
1.,0.866025403784439,1.,0.866025403784439,1.,0.866025403784439,1.))
REPRESENTATION_ITEM('')
);
#4243=(
BOUNDED_CURVE()
B_SPLINE_CURVE(2,(#369264,#369265,#369266,#369267,#369268,#369269,#369270,
#369271,#369272,#369273,#369274,#369275,#369276),.UNSPECIFIED.,.F.,.F.)
B_SPLINE_CURVE_WITH_KNOTS((3,2,2,2,2,2,3),(0.309384940975409,0.318760242217088,
0.328135543458767,0.337510844700446,0.346886145942126,0.356261447183805,
0.365636748425484),.UNSPECIFIED.)
CURVE()
GEOMETRIC_REPRESENTATION_ITEM()
RATIONAL_B_SPLINE_CURVE((1.,0.866025403784439,1.,0.866025403784439,1.,0.866025403784439,
1.,0.866025403784439,1.,0.866025403784439,1.,0.866025403784439,1.))
REPRESENTATION_ITEM('')
);
#4244=(
BOUNDED_CURVE()
B_SPLINE_CURVE(2,(#369281,#369282,#369283,#369284,#369285,#369286,#369287,
#369288,#369289,#369290,#369291,#369292,#369293),.UNSPECIFIED.,.F.,.F.)
B_SPLINE_CURVE_WITH_KNOTS((3,2,2,2,2,2,3),(0.25313309376769,0.262508393536863,
0.271883693306036,0.28125899307521,0.290634292844383,0.300009592613556,
0.309384892382729),.UNSPECIFIED.)
CURVE()
GEOMETRIC_REPRESENTATION_ITEM()
RATIONAL_B_SPLINE_CURVE((1.,0.866025403784439,1.,0.866025403784439,1.,0.866025403784439,
1.,0.866025403784439,1.,0.866025403784439,1.,0.866025403784439,1.))
REPRESENTATION_ITEM('')
);
#4245=(
BOUNDED_CURVE()
B_SPLINE_CURVE(2,(#369294,#369295,#369296,#369297,#369298,#369299,#369300,
#369301,#369302,#369303,#369304,#369305,#369306),.UNSPECIFIED.,.F.,.F.)
B_SPLINE_CURVE_WITH_KNOTS((3,2,2,2,2,2,3),(0.253133133525335,0.262508434767014,
0.271883736008693,0.281259037250372,0.290634338492051,0.30000963973373,
0.309384940975409),.UNSPECIFIED.)
CURVE()
GEOMETRIC_REPRESENTATION_ITEM()
RATIONAL_B_SPLINE_CURVE((1.,0.866025403784439,1.,0.866025403784439,1.,0.866025403784439,
1.,0.866025403784439,1.,0.866025403784439,1.,0.866025403784439,1.))
REPRESENTATION_ITEM('')
);
#4246=(
BOUNDED_CURVE()
B_SPLINE_CURVE(2,(#369311,#369312,#369313,#369314,#369315,#369316,#369317,
#369318,#369319,#369320,#369321,#369322,#369323),.UNSPECIFIED.,.F.,.F.)
B_SPLINE_CURVE_WITH_KNOTS((3,2,2,2,2,2,3),(0.196881295152651,0.206256594921824,
0.215631894690997,0.22500719446017,0.234382494229343,0.243757793998517,
0.25313309376769),.UNSPECIFIED.)
CURVE()
GEOMETRIC_REPRESENTATION_ITEM()
RATIONAL_B_SPLINE_CURVE((1.,0.866025403784439,1.,0.866025403784439,1.,0.866025403784439,
1.,0.866025403784439,1.,0.866025403784439,1.,0.866025403784439,1.))
REPRESENTATION_ITEM('')
);
#4247=(
BOUNDED_CURVE()
B_SPLINE_CURVE(2,(#369324,#369325,#369326,#369327,#369328,#369329,#369330,
#369331,#369332,#369333,#369334,#369335,#369336),.UNSPECIFIED.,.F.,.F.)
B_SPLINE_CURVE_WITH_KNOTS((3,2,2,2,2,2,3),(0.19688132607526,0.20625662731694,
0.215631928558619,0.225007229800298,0.234382531041977,0.243757832283656,
0.253133133525335),.UNSPECIFIED.)
CURVE()
GEOMETRIC_REPRESENTATION_ITEM()
RATIONAL_B_SPLINE_CURVE((1.,0.866025403784439,1.,0.866025403784439,1.,0.866025403784439,
1.,0.866025403784439,1.,0.866025403784439,1.,0.866025403784439,1.))
REPRESENTATION_ITEM('')
);
#4248=(
BOUNDED_CURVE()
B_SPLINE_CURVE(2,(#369341,#369342,#369343,#369344,#369345,#369346,#369347,
#369348,#369349,#369350,#369351,#369352,#369353),.UNSPECIFIED.,.F.,.F.)
B_SPLINE_CURVE_WITH_KNOTS((3,2,2,2,2,2,3),(0.140629496537611,0.150004796306785,
0.159380096075958,0.168755395845131,0.178130695614304,0.187505995383477,
0.196881295152651),.UNSPECIFIED.)
CURVE()
GEOMETRIC_REPRESENTATION_ITEM()
RATIONAL_B_SPLINE_CURVE((1.,0.866025403784439,1.,0.866025403784439,1.,0.866025403784439,
1.,0.866025403784439,1.,0.866025403784439,1.,0.866025403784439,1.))
REPRESENTATION_ITEM('')
);
#4249=(
BOUNDED_CURVE()
B_SPLINE_CURVE(2,(#369354,#369355,#369356,#369357,#369358,#369359,#369360,
#369361,#369362,#369363,#369364,#369365,#369366),.UNSPECIFIED.,.F.,.F.)
B_SPLINE_CURVE_WITH_KNOTS((3,2,2,2,2,2,3),(0.140629518625186,0.150004819866865,
0.159380121108544,0.168755422350223,0.178130723591902,0.187506024833581,
0.19688132607526),.UNSPECIFIED.)
CURVE()
GEOMETRIC_REPRESENTATION_ITEM()
RATIONAL_B_SPLINE_CURVE((1.,0.866025403784439,1.,0.866025403784439,1.,0.866025403784439,
1.,0.866025403784439,1.,0.866025403784439,1.,0.866025403784439,1.))
REPRESENTATION_ITEM('')
);
#4250=(
BOUNDED_CURVE()
B_SPLINE_CURVE(2,(#369371,#369372,#369373,#369374,#369375,#369376,#369377,
#369378,#369379,#369380,#369381,#369382,#369383),.UNSPECIFIED.,.F.,.F.)
B_SPLINE_CURVE_WITH_KNOTS((3,2,2,2,2,2,3),(0.0843776979225721,0.0937529976917453,
0.103128297460919,0.112503597230092,0.121878896999265,0.131254196768438,
0.140629496537611),.UNSPECIFIED.)
CURVE()
GEOMETRIC_REPRESENTATION_ITEM()
RATIONAL_B_SPLINE_CURVE((1.,0.866025403784439,1.,0.866025403784439,1.,0.866025403784439,
1.,0.866025403784439,1.,0.866025403784439,1.,0.866025403784439,1.))
REPRESENTATION_ITEM('')
);
#4251=(
BOUNDED_CURVE()
B_SPLINE_CURVE(2,(#369384,#369385,#369386,#369387,#369388,#369389,#369390,
#369391,#369392,#369393,#369394,#369395,#369396),.UNSPECIFIED.,.F.,.F.)
B_SPLINE_CURVE_WITH_KNOTS((3,2,2,2,2,2,3),(0.0843777111751116,0.0937530124167907,
0.10312831365847,0.112503614900149,0.121878916141828,0.131254217383507,
0.140629518625186),.UNSPECIFIED.)
CURVE()
GEOMETRIC_REPRESENTATION_ITEM()
RATIONAL_B_SPLINE_CURVE((1.,0.866025403784439,1.,0.866025403784439,1.,0.866025403784439,
1.,0.866025403784439,1.,0.866025403784439,1.,0.866025403784439,1.))
REPRESENTATION_ITEM('')
);
#4252=(
BOUNDED_CURVE()
B_SPLINE_CURVE(2,(#369403,#369404,#369405,#369406,#369407,#369408,#369409,
#369410,#369411,#369412,#369413,#369414,#369415),.UNSPECIFIED.,.F.,.F.)
B_SPLINE_CURVE_WITH_KNOTS((3,2,2,2,2,2,3),(0.033715912765314,0.0375011990767061,
0.0468764988458793,0.0562517986150525,0.0656270983842257,0.0750023981533989,
0.0843776979225721),.UNSPECIFIED.)
CURVE()
GEOMETRIC_REPRESENTATION_ITEM()
RATIONAL_B_SPLINE_CURVE((0.93549495027976,0.945907627743645,1.,0.866025403784439,
1.,0.866025403784439,1.,0.866025403784439,1.,0.866025403784439,1.,0.866025403784439,
1.))
REPRESENTATION_ITEM('')
);
#4253=(
BOUNDED_CURVE()
B_SPLINE_CURVE(2,(#369416,#369417,#369418,#369419,#369420,#369421,#369422,
#369423,#369424,#369425,#369426,#369427,#369428),.UNSPECIFIED.,.F.,.F.)
B_SPLINE_CURVE_WITH_KNOTS((3,2,2,2,2,2,3),(0.0281259037250372,0.0375012049667163,
0.0468765062083953,0.0562518074500744,0.0656271086917535,0.0750024099334325,
0.0843777111751116),.UNSPECIFIED.)
CURVE()
GEOMETRIC_REPRESENTATION_ITEM()
RATIONAL_B_SPLINE_CURVE((1.,0.866025403784439,1.,0.866025403784439,1.,0.866025403784439,
1.,0.866025403784439,1.,0.866025403784439,1.,0.866025403784439,1.))
REPRESENTATION_ITEM('')
);
#4254=(
BOUNDED_CURVE()
B_SPLINE_CURVE(2,(#370584,#370585,#370586),.UNSPECIFIED.,.F.,.F.)
B_SPLINE_CURVE_WITH_KNOTS((3,3),(0.120361405182823,0.287808339382405),
 .UNSPECIFIED.)
CURVE()
GEOMETRIC_REPRESENTATION_ITEM()
RATIONAL_B_SPLINE_CURVE((1.61880215351743,1.86923171819516,1.61880215351743))
REPRESENTATION_ITEM('')
);
#4255=(
BOUNDED_CURVE()
B_SPLINE_CURVE(2,(#370694,#370695,#370696),.UNSPECIFIED.,.F.,.F.)
B_SPLINE_CURVE_WITH_KNOTS((3,3),(0.120361405182824,0.287808339382406),
 .UNSPECIFIED.)
CURVE()
GEOMETRIC_REPRESENTATION_ITEM()
RATIONAL_B_SPLINE_CURVE((1.61880215351743,1.86923171819516,1.61880215351743))
REPRESENTATION_ITEM('')
);
#4256=(
BOUNDED_CURVE()
B_SPLINE_CURVE(2,(#370698,#370699,#370700),.UNSPECIFIED.,.F.,.F.)
B_SPLINE_CURVE_WITH_KNOTS((3,3),(0.120361405182823,0.287808339382407),
 .UNSPECIFIED.)
CURVE()
GEOMETRIC_REPRESENTATION_ITEM()
RATIONAL_B_SPLINE_CURVE((1.61880215351743,1.86923171819516,1.61880215351743))
REPRESENTATION_ITEM('')
);
#4257=(
BOUNDED_CURVE()
B_SPLINE_CURVE(2,(#370702,#370703,#370704),.UNSPECIFIED.,.F.,.F.)
B_SPLINE_CURVE_WITH_KNOTS((3,3),(0.120361405182823,0.287808339382406),
 .UNSPECIFIED.)
CURVE()
GEOMETRIC_REPRESENTATION_ITEM()
RATIONAL_B_SPLINE_CURVE((1.61880215351743,1.86923171819516,1.61880215351743))
REPRESENTATION_ITEM('')
);
#4258=(
BOUNDED_CURVE()
B_SPLINE_CURVE(2,(#370706,#370707,#370708),.UNSPECIFIED.,.F.,.F.)
B_SPLINE_CURVE_WITH_KNOTS((3,3),(0.120361405182824,0.287808339382405),
 .UNSPECIFIED.)
CURVE()
GEOMETRIC_REPRESENTATION_ITEM()
RATIONAL_B_SPLINE_CURVE((1.61880215351743,1.86923171819515,1.61880215351743))
REPRESENTATION_ITEM('')
);
#4259=(
BOUNDED_CURVE()
B_SPLINE_CURVE(2,(#370710,#370711,#370712),.UNSPECIFIED.,.F.,.F.)
B_SPLINE_CURVE_WITH_KNOTS((3,3),(0.120361405182823,0.287808339382406),
 .UNSPECIFIED.)
CURVE()
GEOMETRIC_REPRESENTATION_ITEM()
RATIONAL_B_SPLINE_CURVE((1.61880215351743,1.86923171819516,1.61880215351743))
REPRESENTATION_ITEM('')
);
#4260=(
BOUNDED_CURVE()
B_SPLINE_CURVE(2,(#371174,#371175,#371176),.UNSPECIFIED.,.F.,.F.)
B_SPLINE_CURVE_WITH_KNOTS((3,3),(0.0266276333531501,0.0281259037250372),
 .UNSPECIFIED.)
CURVE()
GEOMETRIC_REPRESENTATION_ITEM()
RATIONAL_B_SPLINE_CURVE((0.964022189566802,0.978589470042526,1.))
REPRESENTATION_ITEM('')
);
#4418=SHAPE_REPRESENTATION_RELATIONSHIP('SRR','None',#459344,#4439);
#4439=ADVANCED_BREP_SHAPE_REPRESENTATION('',(#4486),#459233);
#4486=MANIFOLD_SOLID_BREP('Body1',#94664);
#4606=STYLED_ITEM('',(#459533),#4486);
#4895=CONICAL_SURFACE('',#99351,1.25000000000001,0.78539816339745);
#4896=CONICAL_SURFACE('',#99356,0.866025403784441,0.78539816339745);
#4897=CONICAL_SURFACE('',#99361,2.5,0.785398163397448);
#4898=CONICAL_SURFACE('',#99371,0.866025403784441,0.78539816339745);
#4899=CONICAL_SURFACE('',#99372,0.866025403784441,0.78539816339745);
#4900=CONICAL_SURFACE('',#99373,0.866025403784441,0.78539816339745);
#4901=CONICAL_SURFACE('',#99374,0.866025403784441,0.78539816339745);
#4902=CONICAL_SURFACE('',#99375,0.866025403784441,0.78539816339745);
#5225=FACE_BOUND('',#14454,.T.);
#5716=PLANE('',#99364);
#5717=PLANE('',#99370);
#5718=PLANE('',#99376);
#5719=PLANE('',#99377);
#5720=PLANE('',#99378);
#5721=PLANE('',#99379);
#5722=PLANE('',#99380);
#5723=PLANE('',#99381);
#5724=PLANE('',#99382);
#5725=PLANE('',#99383);
#8499=FACE_OUTER_BOUND('',#14419,.T.);
#8500=FACE_OUTER_BOUND('',#14420,.T.);
#8501=FACE_OUTER_BOUND('',#14421,.T.);
#8502=FACE_OUTER_BOUND('',#14422,.T.);
#8503=FACE_OUTER_BOUND('',#14423,.T.);
#8504=FACE_OUTER_BOUND('',#14424,.T.);
#8505=FACE_OUTER_BOUND('',#14425,.T.);
#8506=FACE_OUTER_BOUND('',#14426,.T.);
#8507=FACE_OUTER_BOUND('',#14427,.T.);
#8508=FACE_OUTER_BOUND('',#14428,.T.);
#8509=FACE_OUTER_BOUND('',#14429,.T.);
#8510=FACE_OUTER_BOUND('',#14430,.T.);
#8511=FACE_OUTER_BOUND('',#14431,.T.);
#8512=FACE_OUTER_BOUND('',#14432,.T.);
#8513=FACE_OUTER_BOUND('',#14433,.T.);
#8514=FACE_OUTER_BOUND('',#14434,.T.);
#8515=FACE_OUTER_BOUND('',#14435,.T.);
#8516=FACE_OUTER_BOUND('',#14436,.T.);
#8517=FACE_OUTER_BOUND('',#14437,.T.);
#8518=FACE_OUTER_BOUND('',#14438,.T.);
#8519=FACE_OUTER_BOUND('',#14439,.T.);
#8520=FACE_OUTER_BOUND('',#14440,.T.);
#8521=FACE_OUTER_BOUND('',#14441,.T.);
#8522=FACE_OUTER_BOUND('',#14442,.T.);
#8523=FACE_OUTER_BOUND('',#14443,.T.);
#8524=FACE_OUTER_BOUND('',#14444,.T.);
#8525=FACE_OUTER_BOUND('',#14445,.T.);
#8526=FACE_OUTER_BOUND('',#14446,.T.);
#8527=FACE_OUTER_BOUND('',#14447,.T.);
#8528=FACE_OUTER_BOUND('',#14448,.T.);
#8529=FACE_OUTER_BOUND('',#14449,.T.);
#8530=FACE_OUTER_BOUND('',#14450,.T.);
#8531=FACE_OUTER_BOUND('',#14451,.T.);
#8532=FACE_OUTER_BOUND('',#14452,.T.);
#8533=FACE_OUTER_BOUND('',#14453,.T.);
#8534=FACE_OUTER_BOUND('',#14455,.T.);
#8535=FACE_OUTER_BOUND('',#14456,.T.);
#8536=FACE_OUTER_BOUND('',#14457,.T.);
#8537=FACE_OUTER_BOUND('',#14458,.T.);
#8538=FACE_OUTER_BOUND('',#14459,.T.);
#8539=FACE_OUTER_BOUND('',#14460,.T.);
#8540=FACE_OUTER_BOUND('',#14461,.T.);
#8541=FACE_OUTER_BOUND('',#14462,.T.);
#8542=FACE_OUTER_BOUND('',#14463,.T.);
#8543=FACE_OUTER_BOUND('',#14464,.T.);
#8544=FACE_OUTER_BOUND('',#14465,.T.);
#8545=FACE_OUTER_BOUND('',#14466,.T.);
#8546=FACE_OUTER_BOUND('',#14467,.T.);
#8547=FACE_OUTER_BOUND('',#14468,.T.);
#8548=FACE_OUTER_BOUND('',#14469,.T.);
#8549=FACE_OUTER_BOUND('',#14470,.T.);
#8550=FACE_OUTER_BOUND('',#14471,.T.);
#14419=EDGE_LOOP('',(#69656,#69657,#69658,#69659));
#14420=EDGE_LOOP('',(#69660,#69661,#69662,#69663));
#14421=EDGE_LOOP('',(#69664,#69665,#69666,#69667));
#14422=EDGE_LOOP('',(#69668,#69669,#69670,#69671));
#14423=EDGE_LOOP('',(#69672,#69673,#69674,#69675));
#14424=EDGE_LOOP('',(#69676,#69677,#69678,#69679));
#14425=EDGE_LOOP('',(#69680,#69681,#69682,#69683));
#14426=EDGE_LOOP('',(#69684,#69685,#69686,#69687));
#14427=EDGE_LOOP('',(#69688,#69689,#69690,#69691));
#14428=EDGE_LOOP('',(#69692,#69693,#69694,#69695));
#14429=EDGE_LOOP('',(#69696,#69697,#69698,#69699));
#14430=EDGE_LOOP('',(#69700,#69701,#69702,#69703));
#14431=EDGE_LOOP('',(#69704,#69705,#69706,#69707));
#14432=EDGE_LOOP('',(#69708,#69709,#69710,#69711));
#14433=EDGE_LOOP('',(#69712,#69713,#69714,#69715,#69716));
#14434=EDGE_LOOP('',(#69717,#69718,#69719,#69720));
#14435=EDGE_LOOP('',(#69721,#69722,#69723,#69724));
#14436=EDGE_LOOP('',(#69725,#69726,#69727,#69728));
#14437=EDGE_LOOP('',(#69729,#69730,#69731,#69732));
#14438=EDGE_LOOP('',(#69733,#69734,#69735,#69736));
#14439=EDGE_LOOP('',(#69737,#69738,#69739,#69740));
#14440=EDGE_LOOP('',(#69741,#69742,#69743,#69744));
#14441=EDGE_LOOP('',(#69745,#69746,#69747,#69748));
#14442=EDGE_LOOP('',(#69749,#69750,#69751,#69752));
#14443=EDGE_LOOP('',(#69753,#69754,#69755,#69756));
#14444=EDGE_LOOP('',(#69757,#69758,#69759,#69760));
#14445=EDGE_LOOP('',(#69761,#69762,#69763,#69764));
#14446=EDGE_LOOP('',(#69765,#69766,#69767,#69768));
#14447=EDGE_LOOP('',(#69769,#69770,#69771,#69772));
#14448=EDGE_LOOP('',(#69773,#69774,#69775,#69776,#69777,#69778,#69779,#69780,
#69781));
#14449=EDGE_LOOP('',(#69782,#69783,#69784,#69785));
#14450=EDGE_LOOP('',(#69786,#69787));
#14451=EDGE_LOOP('',(#69788,#69789,#69790,#69791));
#14452=EDGE_LOOP('',(#69792,#69793,#69794,#69795,#69796,#69797,#69798,#69799));
#14453=EDGE_LOOP('',(#69800));
#14454=EDGE_LOOP('',(#69801,#69802,#69803,#69804,#69805,#69806));
#14455=EDGE_LOOP('',(#69807,#69808,#69809,#69810,#69811));
#14456=EDGE_LOOP('',(#69812,#69813));
#14457=EDGE_LOOP('',(#69814,#69815));
#14458=EDGE_LOOP('',(#69816,#69817));
#14459=EDGE_LOOP('',(#69818,#69819));
#14460=EDGE_LOOP('',(#69820,#69821));
#14461=EDGE_LOOP('',(#69822,#69823,#69824,#69825,#69826,#69827));
#14462=EDGE_LOOP('',(#69828,#69829,#69830,#69831));
#14463=EDGE_LOOP('',(#69832,#69833,#69834,#69835));
#14464=EDGE_LOOP('',(#69836,#69837,#69838,#69839));
#14465=EDGE_LOOP('',(#69840,#69841,#69842,#69843));
#14466=EDGE_LOOP('',(#69844,#69845,#69846,#69847));
#14467=EDGE_LOOP('',(#69848,#69849,#69850,#69851));
#14468=EDGE_LOOP('',(#69852));
#14469=EDGE_LOOP('',(#69853,#69854,#69855,#69856,#69857,#69858,#69859,#69860,
#69861,#69862,#69863,#69864,#69865,#69866,#69867,#69868,#69869,#69870,#69871,
#69872,#69873,#69874,#69875,#69876,#69877,#69878,#69879,#69880,#69881,#69882,
#69883,#69884,#69885,#69886));
#14470=EDGE_LOOP('',(#69887,#69888,#69889));
#14471=EDGE_LOOP('',(#69890,#69891,#69892,#69893,#69894,#69895,#69896,#69897,
#69898,#69899,#69900,#69901,#69902,#69903,#69904,#69905,#69906,#69907,#69908,
#69909,#69910,#69911,#69912,#69913,#69914,#69915,#69916,#69917,#69918,#69919,
#69920,#69921,#69922,#69923));
#20590=CIRCLE('',#99320,0.957716426222737);
#20591=CIRCLE('',#99335,0.957716426224497);
#20592=CIRCLE('',#99337,1.25000000000001);
#20593=CIRCLE('',#99352,0.957716426224497);
#20594=CIRCLE('',#99353,0.912499999999999);
#20595=CIRCLE('',#99355,1.25000000000001);
#20596=CIRCLE('',#99357,0.866025403784441);
#20597=CIRCLE('',#99359,2.5);
#20598=CIRCLE('',#99360,2.5);
#20599=CIRCLE('',#99362,1.075);
#20600=CIRCLE('',#99363,1.075);
#20601=CIRCLE('',#99365,0.866025403784441);
#20602=CIRCLE('',#99366,0.866025403784441);
#20603=CIRCLE('',#99367,0.866025403784441);
#20604=CIRCLE('',#99368,0.866025403784441);
#20605=CIRCLE('',#99369,0.866025403784441);
#24674=B_SPLINE_CURVE_WITH_KNOTS('',3,(#369434,#369435,#369436,#369437,
#369438,#369439,#369440,#369441,#369442,#369443,#369444,#369445,#369446,
#369447,#369448,#369449),.UNSPECIFIED.,.F.,.F.,(4,2,2,2,2,2,2,4),(-0.297225196933553,
-0.280367832092781,-0.230062986451411,-0.181680660100882,-0.132941021745363,
-0.0832685681768193,-0.0412377906385104,-1.00000019265245E-6),
 .UNSPECIFIED.);
#24675=B_SPLINE_CURVE_WITH_KNOTS('',3,(#369452,#369453,#369454,#369455,
#369456,#369457,#369458,#369459,#369460,#369461,#369462,#369463),
 .UNSPECIFIED.,.F.,.F.,(4,2,2,2,2,4),(-11.0969330641696,-11.0506498768724,
-11.0060400646789,-10.9574795152701,-10.9078210422652,-10.9002432379435),
 .UNSPECIFIED.);
#24676=B_SPLINE_CURVE_WITH_KNOTS('',3,(#369468,#369469,#369470,#369471,
#369472,#369473,#369474,#369475,#369476,#369477,#369478,#369479,#369480,
#369481,#369482,#369483,#369484,#369485,#369486,#369487,#369488,#369489,
#369490,#369491,#369492,#369493,#369494,#369495,#369496,#369497,#369498,
#369499,#369500,#369501,#369502,#369503),.UNSPECIFIED.,.F.,.F.,(4,2,2,2,
2,2,2,2,2,2,2,2,2,2,2,2,2,4),(-1.08629683604889,-1.06212709216772,-1.01217701512861,
-0.964116528793942,-0.914651515668606,-0.865348804113709,-0.817791776405739,
-0.768003359154763,-0.719235136420373,-0.671389710240228,-0.621277273749783,
-0.573069866056996,-0.524011681351026,-0.474536688662335,-0.426872955991605,
-0.377053394668109,-0.328108386382734,-0.297225196933553),.UNSPECIFIED.);
#24677=B_SPLINE_CURVE_WITH_KNOTS('',3,(#369504,#369505,#369506,#369507,
#369508,#369509,#369510,#369511,#369512,#369513,#369514,#369515,#369516,
#369517,#369518,#369519,#369520,#369521,#369522,#369523,#369524,#369525,
#369526,#369527,#369528,#369529,#369530,#369531,#369532,#369533,#369534,
#369535,#369536,#369537,#369538,#369539),.UNSPECIFIED.,.F.,.F.,(4,2,2,2,
2,2,2,2,2,2,2,2,2,2,2,2,2,4),(-10.9002432379435,-10.8604065333801,-10.8113104443889,
-10.761713814826,-10.7138417906742,-10.6640923927412,-10.616045003083,-10.5676123012695,
-10.5179413964518,-10.470506852643,-10.4215353486384,-10.371439901378,-10.3236642057133,
-10.2740225073813,-10.2256879132737,-10.1773476975794,-10.1276391307857,
-10.1132239534235),.UNSPECIFIED.);
#24678=B_SPLINE_CURVE_WITH_KNOTS('',3,(#369544,#369545,#369546,#369547,
#369548,#369549,#369550,#369551,#369552,#369553,#369554,#369555,#369556,
#369557,#369558,#369559,#369560,#369561,#369562,#369563,#369564,#369565,
#369566,#369567,#369568,#369569,#369570,#369571,#369572,#369573,#369574,
#369575,#369576,#369577,#369578,#369579),.UNSPECIFIED.,.F.,.F.,(4,2,2,2,
2,2,2,2,2,2,2,2,2,2,2,2,2,4),(-1.87536861874309,-1.84355584199448,-1.79384949462906,
-1.74600741502996,-1.69621082068226,-1.64716056762169,-1.59957435410145,
-1.5497648282856,-1.5012562446633,-1.45296588180679,-1.40314413691098,-1.35519906350488,
-1.305259866274,-1.25610014245001,-1.20856696990882,-1.15878121320228,-1.11015973495678,
-1.08629683604889),.UNSPECIFIED.);
#24679=B_SPLINE_CURVE_WITH_KNOTS('',3,(#369580,#369581,#369582,#369583,
#369584,#369585,#369586,#369587,#369588,#369589,#369590,#369591,#369592,
#369593,#369594,#369595,#369596,#369597,#369598,#369599,#369600,#369601,
#369602,#369603,#369604,#369605,#369606,#369607,#369608,#369609,#369610,
#369611,#369612,#369613,#369614,#369615),.UNSPECIFIED.,.F.,.F.,(4,2,2,2,
2,2,2,2,2,2,2,2,2,2,2,2,2,4),(-10.1132239534235,-10.0801144057446,-10.0312319726685,
-9.98154103730301,-9.93385667477381,-9.88431791432676,-9.83555841579789,
-9.78730128208498,-9.73712994715777,-9.68943338837994,-9.64061521762979,
-9.59087875638848,-9.54332419146615,-9.49397528474752,-9.44486869631985,
-9.3967780067164,-9.34679000923077,-9.3251899560265),.UNSPECIFIED.);
#24680=B_SPLINE_CURVE_WITH_KNOTS('',3,(#369620,#369621,#369622,#369623,
#369624,#369625,#369626,#369627,#369628,#369629,#369630,#369631,#369632,
#369633,#369634,#369635,#369636,#369637,#369638,#369639,#369640,#369641,
#369642,#369643,#369644,#369645,#369646,#369647,#369648,#369649,#369650,
#369651,#369652,#369653,#369654,#369655),.UNSPECIFIED.,.F.,.F.,(4,2,2,2,
2,2,2,2,2,2,2,2,2,2,2,2,2,4),(-2.66450830210884,-2.62523893706397,-2.57591415214878,
-2.52835492082748,-2.47857795237277,-2.42978650601587,-2.38198894395603,
-2.33185002481024,-2.28361946775828,-2.23466059104454,-2.18515729676512,
-2.1374720120089,-2.08765685324303,-2.03868217100641,-1.99096903863913,
-1.94063103897361,-1.89221929222858,-1.87536861874309),.UNSPECIFIED.);
#24681=B_SPLINE_CURVE_WITH_KNOTS('',3,(#369656,#369657,#369658,#369659,
#369660,#369661,#369662,#369663,#369664,#369665,#369666,#369667,#369668,
#369669,#369670,#369671,#369672,#369673,#369674,#369675,#369676,#369677,
#369678,#369679,#369680,#369681,#369682,#369683,#369684,#369685,#369686,
#369687,#369688,#369689,#369690,#369691),.UNSPECIFIED.,.F.,.F.,(4,2,2,2,
2,2,2,2,2,2,2,2,2,2,2,2,2,4),(-9.3251899560265,-9.29896232620477,-9.25031178750326,
-9.20059733433329,-9.15312351256986,-9.10393801333592,-9.05440164539032,
-9.00644825470644,-8.95661223118013,-8.90857392265958,-8.86005981037984,
-8.81033962393501,-8.76286474277573,-8.71381206706934,-8.66378663798527,
-8.61593806564963,-8.56621891848283,-8.53743262087695),.UNSPECIFIED.);
#24682=B_SPLINE_CURVE_WITH_KNOTS('',3,(#369696,#369697,#369698,#369699,
#369700,#369701,#369702,#369703,#369704,#369705,#369706,#369707,#369708,
#369709,#369710,#369711,#369712,#369713,#369714,#369715,#369716,#369717,
#369718,#369719,#369720,#369721,#369722,#369723,#369724,#369725,#369726,
#369727,#369728,#369729,#369730,#369731),.UNSPECIFIED.,.F.,.F.,(4,2,2,2,
2,2,2,2,2,2,2,2,2,2,2,2,2,4),(-3.45311041785451,-3.40640578800035,-3.35734889527748,
-3.30979687791647,-3.26001136181265,-3.21149516431656,-3.16328629585956,
-3.11345375633878,-3.06550007523919,-3.01569323829511,-2.96651867048036,
-2.91900255270055,-2.86923473474433,-2.8205974011257,-2.77263121805615,
-2.72266205646393,-2.6745852915141,-2.66450830210884),.UNSPECIFIED.);
#24683=B_SPLINE_CURVE_WITH_KNOTS('',3,(#369732,#369733,#369734,#369735,
#369736,#369737,#369738,#369739,#369740,#369741,#369742,#369743,#369744,
#369745,#369746,#369747,#369748,#369749,#369750,#369751,#369752,#369753,
#369754,#369755,#369756,#369757,#369758,#369759,#369760,#369761,#369762,
#369763,#369764,#369765,#369766,#369767),.UNSPECIFIED.,.F.,.F.,(4,2,2,2,
2,2,2,2,2,2,2,2,2,2,2,2,2,4),(-8.53743262087695,-8.51790557886756,-8.4694930188994,
-8.41974122096977,-8.37219191612705,-8.32323738821537,-8.27350131454077,
-8.22574932274126,-8.17613872282825,-8.12742281473662,-8.07909951276689,
-8.0288568753523,-7.98115537034797,-7.9322702522769,-7.8825002114564,-7.83489172319436,
-7.7854767277125,-7.74885616038243),.UNSPECIFIED.);
#24684=B_SPLINE_CURVE_WITH_KNOTS('',3,(#369772,#369773,#369774,#369775,
#369776,#369777,#369778,#369779,#369780,#369781,#369782,#369783,#369784,
#369785,#369786,#369787,#369788,#369789,#369790,#369791,#369792,#369793,
#369794,#369795,#369796,#369797,#369798,#369799,#369800,#369801,#369802,
#369803,#369804,#369805,#369806,#369807,#369808,#369809),.UNSPECIFIED.,
 .F.,.F.,(4,2,2,2,2,2,2,2,2,2,2,2,2,2,2,2,2,2,4),(-4.24192213155039,-4.23809792147632,
-4.18836234856388,-4.13957498951885,-4.09185274799052,-4.04171529566761,
-3.9934886596208,-3.94465978359765,-3.89515592670361,-3.84747283207717,
-3.79769147839944,-3.74871439112587,-3.7010548294868,-3.65071175267311,
-3.60229775019791,-3.55373929331727,-3.50402693278433,-3.45618073503253,
-3.45311041785451),.UNSPECIFIED.);
#24685=B_SPLINE_CURVE_WITH_KNOTS('',3,(#369810,#369811,#369812,#369813,
#369814,#369815,#369816,#369817,#369818,#369819,#369820,#369821,#369822,
#369823,#369824,#369825,#369826,#369827,#369828,#369829,#369830,#369831,
#369832,#369833,#369834,#369835,#369836,#369837,#369838,#369839,#369840,
#369841,#369842,#369843,#369844,#369845),.UNSPECIFIED.,.F.,.F.,(4,2,2,2,
2,2,2,2,2,2,2,2,2,2,2,2,2,4),(-7.74885616038243,-7.73643534531436,-7.68828489874703,
-7.63823245858939,-7.59041958736585,-7.54170890559822,-7.49196769011302,
-7.44445938896145,-7.39521440060387,-7.34576049706096,-7.2977545191574,
-7.24786179061972,-7.19985584140599,-7.15128928192139,-7.10154861462626,
-7.05405787738374,-7.00495329873603,-6.96074678199533),.UNSPECIFIED.);
#24686=B_SPLINE_CURVE_WITH_KNOTS('',3,(#369850,#369851,#369852,#369853,
#369854,#369855,#369856,#369857,#369858,#369859,#369860,#369861,#369862,
#369863,#369864,#369865,#369866,#369867,#369868,#369869,#369870,#369871,
#369872,#369873,#369874,#369875,#369876,#369877,#369878,#369879,#369880,
#369881,#369882,#369883,#369884,#369885),.UNSPECIFIED.,.F.,.F.,(4,2,2,2,
2,2,2,2,2,2,2,2,2,2,2,2,2,4),(-5.02972443161939,-5.0187363541838,-4.96900575987408,
-4.92050955509127,-4.87241366245925,-4.82259855136958,-4.77466360731621,
-4.72502503301001,-4.67586344949185,-4.62839019418675,-4.57867076701161,
-4.53004498522224,-4.48217452916704,-4.43221432415173,-4.38414845254951,
-4.33495397914721,-4.28563488367131,-4.24192213155039),.UNSPECIFIED.);
#24687=B_SPLINE_CURVE_WITH_KNOTS('',3,(#369886,#369887,#369888,#369889,
#369890,#369891,#369892,#369893,#369894,#369895,#369896,#369897,#369898,
#369899,#369900,#369901,#369902,#369903,#369904,#369905,#369906,#369907,
#369908,#369909,#369910,#369911,#369912,#369913,#369914,#369915,#369916,
#369917,#369918,#369919,#369920,#369921,#369922,#369923),.UNSPECIFIED.,
 .F.,.F.,(4,2,2,2,2,2,2,2,2,2,2,2,2,2,2,2,2,2,4),(-6.96074678199533,-6.95502152207767,
-6.90527708144643,-6.85655770199055,-6.80874804770292,-6.75868624361776,
-6.71052715808686,-6.66149720058363,-6.61207258246791,-6.56445611871926,
-6.51468173086547,-6.46578683168715,-6.41808529513843,-6.36783220114316,
-6.31949923703344,-6.27079116033409,-6.2211700228527,-6.17340813772743,
-6.17206263548208),.UNSPECIFIED.);
#24688=B_SPLINE_CURVE_WITH_KNOTS('',3,(#369928,#369929,#369930,#369931,
#369932,#369933,#369934,#369935,#369936,#369937,#369938,#369939,#369940,
#369941,#369942,#369943,#369944,#369945,#369946,#369947,#369948,#369949,
#369950,#369951,#369952,#369953,#369954,#369955,#369956,#369957,#369958,
#369959,#369960,#369961,#369962,#369963),.UNSPECIFIED.,.F.,.F.,(4,2,2,2,
2,2,2,2,2,2,2,2,2,2,2,2,2,4),(-5.81829984350504,-5.80046863144242,-5.75023363519347,
-5.70191564674989,-5.65311229785516,-5.60351043799573,-5.55576557565544,
-5.50601560630357,-5.45707070341708,-5.40949261239909,-5.35972528079792,
-5.31132312095601,-5.26294159013347,-5.21323577254684,-5.16539862838024,
-5.11526216484913,-5.06622663267278,-5.02972443161939),.UNSPECIFIED.);
#24689=B_SPLINE_CURVE_WITH_KNOTS('',3,(#369964,#369965,#369966,#369967,
#369968,#369969,#369970,#369971,#369972,#369973,#369974,#369975,#369976,
#369977,#369978,#369979,#369980,#369981,#369982,#369983,#369984,#369985,
#369986,#369987,#369988,#369989,#369990,#369991,#369992,#369993,#369994,
#369995,#369996,#369997,#369998,#369999),.UNSPECIFIED.,.F.,.F.,(4,2,2,2,
2,2,2,2,2,2,2,2,2,2,2,2,2,4),(-6.17206263548208,-6.12366583999162,-6.07470074073969,
-6.02714826734756,-5.97739057213024,-5.92896739037585,-5.88065826419392,
-5.83092771067481,-5.78306843191849,-5.73305506215986,-5.68399039252467,
-5.63650975764823,-5.58678270549522,-5.53825654861325,-5.49022040156367,
-5.44037153355227,-5.39240610619022,-5.38405069970025),.UNSPECIFIED.);
#24690=B_SPLINE_CURVE_WITH_KNOTS('',3,(#370004,#370005,#370006,#370007,
#370008,#370009,#370010,#370011,#370012,#370013,#370014,#370015,#370016,
#370017,#370018,#370019,#370020,#370021,#370022,#370023,#370024,#370025,
#370026,#370027,#370028,#370029,#370030,#370031,#370032,#370033,#370034,
#370035,#370036,#370037,#370038,#370039),.UNSPECIFIED.,.F.,.F.,(4,2,2,2,
2,2,2,2,2,2,2,2,2,2,2,2,2,4),(-6.60703756023774,-6.58187604768098,-6.53197903755641,
-6.48396727026408,-6.43439222014541,-6.38514596147057,-6.3376172967117,
-6.28784666941341,-6.23913583046104,-6.19126067984556,-6.14121030559726,
-6.09305995544669,-6.04391250359479,-5.99450161250507,-5.94688905770524,
-5.89709533587369,-5.84821560509502,-5.81829984350504),.UNSPECIFIED.);
#24691=B_SPLINE_CURVE_WITH_KNOTS('',3,(#370040,#370041,#370042,#370043,
#370044,#370045,#370046,#370047,#370048,#370049,#370050,#370051,#370052,
#370053,#370054,#370055,#370056,#370057,#370058,#370059,#370060,#370061,
#370062,#370063,#370064,#370065,#370066,#370067,#370068,#370069,#370070,
#370071,#370072,#370073,#370074,#370075),.UNSPECIFIED.,.F.,.F.,(4,2,2,2,
2,2,2,2,2,2,2,2,2,2,2,2,2,4),(-5.38405069970025,-5.34288008366044,-5.29368130835127,
-5.24619867625064,-5.19647632389707,-5.14781244101478,-5.09998408356202,
-5.04998193383878,-5.00187799656936,-4.95277901109365,-4.90341570644776,
-4.85584909893607,-4.80610361642015,-4.75727094726801,-4.70957047324575,
-4.65938382194792,-4.61111235420568,-4.59595956437439),.UNSPECIFIED.);
#24692=B_SPLINE_CURVE_WITH_KNOTS('',3,(#370080,#370081,#370082,#370083,
#370084,#370085,#370086,#370087,#370088,#370089,#370090,#370091,#370092,
#370093,#370094,#370095,#370096,#370097,#370098,#370099,#370100,#370101,
#370102,#370103,#370104,#370105,#370106,#370107,#370108,#370109,#370110,
#370111,#370112,#370113,#370114,#370115),.UNSPECIFIED.,.F.,.F.,(4,2,2,2,
2,2,2,2,2,2,2,2,2,2,2,2,2,4),(-7.39570158201985,-7.36254636003036,-7.31362768878039,
-7.26390072255125,-7.21618108953506,-7.16660564252708,-7.11781333282715,
-7.06952057237752,-7.02105052930277,-6.97269388442146,-6.92291523017473,
-6.87500964654849,-6.82494668210698,-6.77583459408507,-6.72830776969244,
-6.67853238433299,-6.62995933898348,-6.60703756023774),.UNSPECIFIED.);
#24693=B_SPLINE_CURVE_WITH_KNOTS('',3,(#370116,#370117,#370118,#370119,
#370120,#370121,#370122,#370123,#370124,#370125,#370126,#370127,#370128,
#370129,#370130,#370131,#370132,#370133,#370134,#370135,#370136,#370137,
#370138,#370139,#370140,#370141,#370142,#370143,#370144,#370145,#370146,
#370147,#370148,#370149,#370150,#370151),.UNSPECIFIED.,.F.,.F.,(4,2,2,2,
2,2,2,2,2,2,2,2,2,2,2,2,2,4),(-4.59595956437439,-4.56235695294563,-4.51280281574693,
-4.46510390240623,-4.41540203036628,-4.36650420699104,-4.31897228058962,
-4.269253079062,-4.22089746757123,-4.17256328077253,-4.12290523769736,-4.07511408620101,
-4.0250270996101,-3.97603865570477,-3.92859432163572,-3.87891176911502,
-3.83046212492628,-3.80838734160697),.UNSPECIFIED.);
#24694=B_SPLINE_CURVE_WITH_KNOTS('',3,(#370156,#370157,#370158,#370159,
#370160,#370161,#370162,#370163,#370164,#370165,#370166,#370167,#370168,
#370169,#370170,#370171,#370172,#370173,#370174,#370175,#370176,#370177,
#370178,#370179,#370180,#370181,#370182,#370183,#370184,#370185,#370186,
#370187,#370188,#370189,#370190,#370191),.UNSPECIFIED.,.F.,.F.,(4,2,2,2,
2,2,2,2,2,2,2,2,2,2,2,2,2,4),(-8.18329352926,-8.14340210893405,-8.09426912520822,
-8.04463960472576,-7.99673177620422,-7.94694511105315,-7.89886443645484,
-7.85039553897279,-7.80068849465037,-7.75321967281652,-7.70421160318344,
-7.654083175026,-7.60627199042295,-7.55659336826637,-7.50822562336118,-7.45984954124163,
-7.41010498272117,-7.39570158201985),.UNSPECIFIED.);
#24695=B_SPLINE_CURVE_WITH_KNOTS('',3,(#370192,#370193,#370194,#370195,
#370196,#370197,#370198,#370199,#370200,#370201,#370202,#370203,#370204,
#370205,#370206,#370207,#370208,#370209,#370210,#370211,#370212,#370213,
#370214,#370215,#370216,#370217,#370218,#370219,#370220,#370221,#370222,
#370223,#370224,#370225,#370226,#370227),.UNSPECIFIED.,.F.,.F.,(4,2,2,2,
2,2,2,2,2,2,2,2,2,2,2,2,2,4),(-3.80838734160697,-3.78241319552622,-3.73264588502551,
-3.68475695452833,-3.63516729185455,-3.58605284696992,-3.53862535621508,
-3.48895390409539,-3.44037473596106,-3.39255087588116,-3.34263853913331,
-3.2946187404684,-3.24547260749217,-3.19620074039827,-3.14870942771508,
-3.09902178513712,-3.05028113183768,-3.02126527915157),.UNSPECIFIED.);
#24696=B_SPLINE_CURVE_WITH_KNOTS('',3,(#370232,#370233,#370234,#370235,
#370236,#370237,#370238,#370239,#370240,#370241,#370242,#370243,#370244,
#370245,#370246,#370247,#370248,#370249,#370250,#370251,#370252,#370253,
#370254,#370255,#370256,#370257,#370258,#370259,#370260,#370261,#370262,
#370263,#370264,#370265,#370266,#370267),.UNSPECIFIED.,.F.,.F.,(4,2,2,2,
2,2,2,2,2,2,2,2,2,2,2,2,2,4),(-8.97097791248705,-8.92371187470672,-8.8742385366992,
-8.82542327411857,-8.77722580886648,-8.72711902037387,-8.67941669194377,
-8.63065883194959,-8.58094855992311,-8.5334381898614,-8.48414871101692,
-8.43496520836685,-8.38692752659352,-8.33699692985527,-8.28914382647278,
-8.24054650130081,-8.19085146033859,-8.18329352926),.UNSPECIFIED.);
#24697=B_SPLINE_CURVE_WITH_KNOTS('',3,(#370268,#370269,#370270,#370271,
#370272,#370273,#370274,#370275,#370276,#370277,#370278,#370279,#370280,
#370281,#370282,#370283,#370284,#370285,#370286,#370287,#370288,#370289,
#370290,#370291,#370292,#370293,#370294,#370295,#370296,#370297,#370298,
#370299,#370300,#370301,#370302,#370303),.UNSPECIFIED.,.F.,.F.,(4,2,2,2,
2,2,2,2,2,2,2,2,2,2,2,2,2,4),(-3.02126527915157,-3.00260516806742,-2.95251569085902,
-2.90433522308815,-2.85555414669426,-2.80609764269441,-2.75846016823742,
-2.70872672337365,-2.6597964690442,-2.61218293988413,-2.56188798012619,
-2.51352027335298,-2.46500914259868,-2.41534428872647,-2.36754382854494,
-2.31781668136951,-2.26880666392932,-2.23313514244992),.UNSPECIFIED.);
#24698=B_SPLINE_CURVE_WITH_KNOTS('',3,(#370308,#370309,#370310,#370311,
#370312,#370313,#370314,#370315,#370316,#370317,#370318,#370319,#370320,
#370321,#370322,#370323,#370324,#370325,#370326,#370327,#370328,#370329,
#370330,#370331,#370332,#370333,#370334,#370335,#370336,#370337,#370338,
#370339,#370340,#370341,#370342,#370343,#370344,#370345),.UNSPECIFIED.,
 .F.,.F.,(4,2,2,2,2,2,2,2,2,2,2,2,2,2,2,2,2,2,4),(-9.75953055606769,-9.75289518479629,
-9.70497206855282,-9.65517152839672,-9.60698210655507,-9.55849670090529,
-9.508738741953,-9.46121175815317,-9.4121858661215,-9.36243877625384,-9.31462252400408,
-9.26494150013379,-9.21639972157875,-9.16801578697161,-9.11770432709358,
-9.07006743064845,-9.02112077880878,-8.97136573631902,-8.97097791248705),
 .UNSPECIFIED.);
#24699=B_SPLINE_CURVE_WITH_KNOTS('',3,(#370346,#370347,#370348,#370349,
#370350,#370351,#370352,#370353,#370354,#370355,#370356,#370357,#370358,
#370359,#370360,#370361,#370362,#370363,#370364,#370365,#370366,#370367,
#370368,#370369,#370370,#370371,#370372,#370373,#370374,#370375,#370376,
#370377,#370378,#370379,#370380,#370381),.UNSPECIFIED.,.F.,.F.,(4,2,2,2,
2,2,2,2,2,2,2,2,2,2,2,2,2,4),(-2.23313514244992,-2.22130041501826,-2.17156272926473,
-2.12309288159397,-2.0749308070373,-2.02514585029162,-1.97723797307212,
-1.92747988450581,-1.87835223712549,-1.83088170783493,-1.78116165238413,
-1.73257071664056,-1.68465096511949,-1.63472944881252,-1.58669854238685,
-1.53740037538244,-1.48812259544505,-1.44532777081289),.UNSPECIFIED.);
#24700=B_SPLINE_CURVE_WITH_KNOTS('',3,(#370386,#370387,#370388,#370389,
#370390,#370391,#370392,#370393,#370394,#370395,#370396,#370397,#370398,
#370399,#370400,#370401,#370402,#370403,#370404,#370405,#370406,#370407,
#370408,#370409,#370410,#370411,#370412,#370413,#370414,#370415,#370416,
#370417,#370418,#370419,#370420,#370421),.UNSPECIFIED.,.F.,.F.,(4,2,2,2,
2,2,2,2,2,2,2,2,2,2,2,2,2,4),(-10.5477144568492,-10.5343257988314,-10.4861277850314,
-10.4360230035294,-10.3882489608822,-10.3394904162225,-10.2897425906394,
-10.2422130277014,-10.1929213240059,-10.143590495231,-10.0955453254922,
-10.0456092788967,-9.99766435067504,-9.94905890957184,-9.89931940611708,
-9.85183049354891,-9.80268801893929,-9.75953055606769),.UNSPECIFIED.);
#24701=B_SPLINE_CURVE_WITH_KNOTS('',3,(#370422,#370423,#370424,#370425,
#370426,#370427,#370428,#370429,#370430,#370431,#370432,#370433,#370434,
#370435,#370436,#370437,#370438,#370439,#370440,#370441,#370442,#370443,
#370444,#370445,#370446,#370447,#370448,#370449,#370450,#370451,#370452,
#370453,#370454,#370455,#370456,#370457,#370458,#370459),.UNSPECIFIED.,
 .F.,.F.,(4,2,2,2,2,2,2,2,2,2,2,2,2,2,2,2,2,2,4),(-1.44532777081289,-1.44060883240002,
-1.39087958066294,-1.34213461919547,-1.2943831702068,-1.24429199807141,
-1.19610739026894,-1.14719616446327,-1.09773999499641,-1.05010013906413,
-1.00033267427764,-0.951404599399516,-0.903737328903778,-0.853447213420372,
-0.805081539111285,-0.756465263702377,-0.706806190913238,-0.659009625901751,
-0.656744776062406),.UNSPECIFIED.);
#24702=B_SPLINE_CURVE_WITH_KNOTS('',3,(#370463,#370464,#370465,#370466,
#370467,#370468,#370469,#370470,#370471,#370472,#370473,#370474),
 .UNSPECIFIED.,.F.,.F.,(4,2,2,2,2,4),(-0.147125121134148,-0.128349501591643,
-0.105314013958521,-0.0783046855556977,-0.042089246328591,-1.00000017627666E-6),
 .UNSPECIFIED.);
#24703=B_SPLINE_CURVE_WITH_KNOTS('',3,(#370476,#370477,#370478,#370479,
#370480,#370481,#370482,#370483,#370484,#370485,#370486,#370487,#370488,
#370489,#370490,#370491,#370492,#370493,#370494,#370495,#370496,#370497,
#370498,#370499),.UNSPECIFIED.,.F.,.F.,(4,2,2,2,2,2,2,2,2,2,2,4),(-1.13468288871823,
-1.0706043934222,-1.00734719961197,-0.908024292964587,-0.805111116080014,
-0.706602531207623,-0.634633508201914,-0.578664318892748,-0.526740212001412,
-0.472667922135714,-0.421519787488127,-0.367202841889784),.UNSPECIFIED.);
#24704=B_SPLINE_CURVE_WITH_KNOTS('',3,(#370503,#370504,#370505,#370506,
#370507,#370508,#370509,#370510,#370511,#370512,#370513,#370514,#370515,
#370516,#370517,#370518,#370519,#370520),.UNSPECIFIED.,.F.,.F.,(4,2,2,2,
2,2,2,2,4),(-0.367202841889784,-0.360788898680035,-0.297043709635829,-0.22884142572636,
-0.166869586833399,-0.11581538945378,-0.0610544135172069,-0.0270530161618892,
-1.00000019448432E-6),.UNSPECIFIED.);
#24705=B_SPLINE_CURVE_WITH_KNOTS('',3,(#370523,#370524,#370525,#370526,
#370527,#370528,#370529,#370530,#370531,#370532,#370533,#370534,#370535,
#370536,#370537,#370538,#370539,#370540,#370541,#370542,#370543,#370544,
#370545,#370546,#370547,#370548,#370549,#370550,#370551,#370552),
 .UNSPECIFIED.,.F.,.F.,(4,2,2,2,2,2,2,2,2,2,2,2,2,2,4),(-0.656744776062406,
-0.609260683930364,-0.560257149562067,-0.51271659362795,-0.462954754241167,
-0.414492365041179,-0.366248708414827,-0.31647438439645,-0.26857495964527,
-0.218684447711158,-0.1695714801609,-0.122083779620549,-0.0723456381913861,
-0.035554498052184,-1.00000012637214E-6),.UNSPECIFIED.);
#24706=B_SPLINE_CURVE_WITH_KNOTS('',3,(#370555,#370556,#370557,#370558,
#370559,#370560,#370561,#370562,#370563,#370564,#370565,#370566,#370567,
#370568,#370569,#370570,#370571,#370572,#370573,#370574,#370575,#370576,
#370577,#370578,#370579,#370580),.UNSPECIFIED.,.F.,.F.,(4,2,2,2,2,2,2,2,
2,2,2,2,4),(-11.1077295770696,-11.0661775997393,-11.0237973371211,-10.9741258386803,
-10.9254829944382,-10.8771047475493,-10.8268019041466,-10.7791148973966,
-10.7301741164739,-10.6803891069329,-10.6327360727518,-10.5832668289047,
-10.5477144568492),.UNSPECIFIED.);
#24707=B_SPLINE_CURVE_WITH_KNOTS('',3,(#370599,#370600,#370601,#370602,
#370603,#370604,#370605,#370606,#370607,#370608,#370609,#370610,#370611,
#370612,#370613,#370614,#370615,#370616,#370617,#370618,#370619,#370620,
#370621,#370622),.UNSPECIFIED.,.F.,.F.,(4,2,2,2,2,2,2,2,2,2,2,4),(-0.370205279453778,
-0.350219365145943,-0.329577799848427,-0.293539528040863,-0.259747571198344,
-0.227982662210344,-0.199662873529425,-0.16494855267263,-0.124437197575316,
-0.0810928930749654,-0.0392683201053638,-9.99999999307111E-7),
 .UNSPECIFIED.);
#24708=B_SPLINE_CURVE_WITH_KNOTS('',3,(#370624,#370625,#370626,#370627,
#370628,#370629,#370630,#370631,#370632,#370633,#370634,#370635,#370636,
#370637,#370638,#370639,#370640,#370641,#370642,#370643,#370644,#370645,
#370646,#370647,#370648,#370649,#370650,#370651,#370652,#370653,#370654,
#370655,#370656,#370657,#370658,#370659,#370660),.UNSPECIFIED.,.F.,.F.,
(4,3,3,3,3,3,3,3,3,3,3,3,4),(2.99491710979115E-14,0.000108371923709533,
0.00021803673379923,0.000304842679092563,0.000415181043997034,0.000525308370927796,
0.000609685358155176,0.000711172109786132,0.000812850073501961,0.000914528037217789,
0.00102917412252272,0.00114325983251636,0.0012193707162804),
 .UNSPECIFIED.);
#24709=B_SPLINE_CURVE_WITH_KNOTS('',3,(#370673,#370674,#370675,#370676,
#370677,#370678,#370679,#370680,#370681,#370682),.UNSPECIFIED.,.F.,.F.,
(4,2,2,2,4),(-0.115181813240965,-0.083642902448367,-0.0518196847902682,
-0.0231633114822182,0.),.UNSPECIFIED.);
#24710=B_SPLINE_CURVE_WITH_KNOTS('',3,(#370683,#370684,#370685,#370686,
#370687,#370688,#370689,#370690,#370691,#370692),.UNSPECIFIED.,.F.,.F.,
(4,2,2,2,4),(-0.0961593141722214,-0.0719589549439694,-0.0481092230513157,
-0.0251497984388369,-1.00000015684776E-6),.UNSPECIFIED.);
#29034=LINE('',#368991,#32836);
#29035=LINE('',#369010,#32837);
#29036=LINE('',#369040,#32838);
#29037=LINE('',#369070,#32839);
#29038=LINE('',#369100,#32840);
#29039=LINE('',#369130,#32841);
#29040=LINE('',#369160,#32842);
#29041=LINE('',#369190,#32843);
#29042=LINE('',#369220,#32844);
#29043=LINE('',#369250,#32845);
#29044=LINE('',#369280,#32846);
#29045=LINE('',#369310,#32847);
#29046=LINE('',#369340,#32848);
#29047=LINE('',#369370,#32849);
#29048=LINE('',#369400,#32850);
#29049=LINE('',#369432,#32851);
#29050=LINE('',#369467,#32852);
#29051=LINE('',#369543,#32853);
#29052=LINE('',#369619,#32854);
#29053=LINE('',#369695,#32855);
#29054=LINE('',#369771,#32856);
#29055=LINE('',#369849,#32857);
#29056=LINE('',#369927,#32858);
#29057=LINE('',#370003,#32859);
#29058=LINE('',#370079,#32860);
#29059=LINE('',#370155,#32861);
#29060=LINE('',#370231,#32862);
#29061=LINE('',#370307,#32863);
#29062=LINE('',#370385,#32864);
#29063=LINE('',#370501,#32865);
#29064=LINE('',#370592,#32866);
#29065=LINE('',#370596,#32867);
#29066=LINE('',#370716,#32868);
#29067=LINE('',#370718,#32869);
#29068=LINE('',#370720,#32870);
#29069=LINE('',#370722,#32871);
#29070=LINE('',#370724,#32872);
#29071=LINE('',#370725,#32873);
#29072=LINE('',#370727,#32874);
#29073=LINE('',#370728,#32875);
#29074=LINE('',#370730,#32876);
#29075=LINE('',#370732,#32877);
#29076=LINE('',#370734,#32878);
#29077=LINE('',#370736,#32879);
#32836=VECTOR('',#116394,0.957716426222737);
#32837=VECTOR('',#116399,0.957716426222737);
#32838=VECTOR('',#116402,0.957716426222737);
#32839=VECTOR('',#116405,0.957716426222737);
#32840=VECTOR('',#116408,0.957716426222737);
#32841=VECTOR('',#116411,0.957716426222737);
#32842=VECTOR('',#116414,0.957716426222737);
#32843=VECTOR('',#116417,0.957716426222737);
#32844=VECTOR('',#116420,0.957716426222737);
#32845=VECTOR('',#116423,0.957716426222737);
#32846=VECTOR('',#116426,0.957716426222737);
#32847=VECTOR('',#116429,0.957716426222737);
#32848=VECTOR('',#116432,0.957716426222737);
#32849=VECTOR('',#116435,0.957716426222737);
#32850=VECTOR('',#116438,0.957716426222737);
#32851=VECTOR('',#116443,1.25000000000001);
#32852=VECTOR('',#116448,1.25000000000001);
#32853=VECTOR('',#116451,1.25000000000001);
#32854=VECTOR('',#116454,1.25000000000001);
#32855=VECTOR('',#116457,1.25000000000001);
#32856=VECTOR('',#116460,1.25000000000001);
#32857=VECTOR('',#116463,1.25000000000001);
#32858=VECTOR('',#116466,1.25000000000001);
#32859=VECTOR('',#116469,1.25000000000001);
#32860=VECTOR('',#116472,1.25000000000001);
#32861=VECTOR('',#116475,1.25000000000001);
#32862=VECTOR('',#116478,1.25000000000001);
#32863=VECTOR('',#116481,1.25000000000001);
#32864=VECTOR('',#116484,1.25000000000001);
#32865=VECTOR('',#116489,1.25000000000001);
#32866=VECTOR('',#116504,2.5);
#32867=VECTOR('',#116509,2.5);
#32868=VECTOR('',#116540,1000.);
#32869=VECTOR('',#116541,1000.);
#32870=VECTOR('',#116542,1000.);
#32871=VECTOR('',#116543,1000.);
#32872=VECTOR('',#116544,1000.);
#32873=VECTOR('',#116545,1000.);
#32874=VECTOR('',#116548,1000.);
#32875=VECTOR('',#116549,1000.);
#32876=VECTOR('',#116552,1000.);
#32877=VECTOR('',#116555,1000.);
#32878=VECTOR('',#116558,1000.);
#32879=VECTOR('',#116561,1000.);
#38431=VERTEX_POINT('',#368989);
#38432=VERTEX_POINT('',#368990);
#38433=VERTEX_POINT('',#368992);
#38434=VERTEX_POINT('',#369000);
#38435=VERTEX_POINT('',#369008);
#38436=VERTEX_POINT('',#369009);
#38437=VERTEX_POINT('',#369038);
#38438=VERTEX_POINT('',#369039);
#38439=VERTEX_POINT('',#369068);
#38440=VERTEX_POINT('',#369069);
#38441=VERTEX_POINT('',#369098);
#38442=VERTEX_POINT('',#369099);
#38443=VERTEX_POINT('',#369128);
#38444=VERTEX_POINT('',#369129);
#38445=VERTEX_POINT('',#369158);
#38446=VERTEX_POINT('',#369159);
#38447=VERTEX_POINT('',#369188);
#38448=VERTEX_POINT('',#369189);
#38449=VERTEX_POINT('',#369218);
#38450=VERTEX_POINT('',#369219);
#38451=VERTEX_POINT('',#369248);
#38452=VERTEX_POINT('',#369249);
#38453=VERTEX_POINT('',#369278);
#38454=VERTEX_POINT('',#369279);
#38455=VERTEX_POINT('',#369308);
#38456=VERTEX_POINT('',#369309);
#38457=VERTEX_POINT('',#369338);
#38458=VERTEX_POINT('',#369339);
#38459=VERTEX_POINT('',#369368);
#38460=VERTEX_POINT('',#369369);
#38461=VERTEX_POINT('',#369398);
#38462=VERTEX_POINT('',#369399);
#38463=VERTEX_POINT('',#369401);
#38464=VERTEX_POINT('',#369430);
#38465=VERTEX_POINT('',#369431);
#38466=VERTEX_POINT('',#369433);
#38467=VERTEX_POINT('',#369450);
#38468=VERTEX_POINT('',#369465);
#38469=VERTEX_POINT('',#369466);
#38470=VERTEX_POINT('',#369541);
#38471=VERTEX_POINT('',#369542);
#38472=VERTEX_POINT('',#369617);
#38473=VERTEX_POINT('',#369618);
#38474=VERTEX_POINT('',#369693);
#38475=VERTEX_POINT('',#369694);
#38476=VERTEX_POINT('',#369769);
#38477=VERTEX_POINT('',#369770);
#38478=VERTEX_POINT('',#369847);
#38479=VERTEX_POINT('',#369848);
#38480=VERTEX_POINT('',#369925);
#38481=VERTEX_POINT('',#369926);
#38482=VERTEX_POINT('',#370001);
#38483=VERTEX_POINT('',#370002);
#38484=VERTEX_POINT('',#370077);
#38485=VERTEX_POINT('',#370078);
#38486=VERTEX_POINT('',#370153);
#38487=VERTEX_POINT('',#370154);
#38488=VERTEX_POINT('',#370229);
#38489=VERTEX_POINT('',#370230);
#38490=VERTEX_POINT('',#370305);
#38491=VERTEX_POINT('',#370306);
#38492=VERTEX_POINT('',#370383);
#38493=VERTEX_POINT('',#370384);
#38494=VERTEX_POINT('',#370461);
#38495=VERTEX_POINT('',#370475);
#38496=VERTEX_POINT('',#370500);
#38497=VERTEX_POINT('',#370522);
#38498=VERTEX_POINT('',#370553);
#38499=VERTEX_POINT('',#370582);
#38500=VERTEX_POINT('',#370583);
#38501=VERTEX_POINT('',#370589);
#38502=VERTEX_POINT('',#370591);
#38503=VERTEX_POINT('',#370595);
#38504=VERTEX_POINT('',#370597);
#38505=VERTEX_POINT('',#370623);
#38506=VERTEX_POINT('',#370663);
#38507=VERTEX_POINT('',#370665);
#38508=VERTEX_POINT('',#370667);
#38509=VERTEX_POINT('',#370669);
#38510=VERTEX_POINT('',#370714);
#38511=VERTEX_POINT('',#370715);
#38512=VERTEX_POINT('',#370717);
#38513=VERTEX_POINT('',#370719);
#38514=VERTEX_POINT('',#370721);
#38515=VERTEX_POINT('',#370723);
#49330=EDGE_CURVE('',#38431,#38432,#29034,.T.);
#49331=EDGE_CURVE('',#38431,#38433,#4224,.T.);
#49332=EDGE_CURVE('',#38433,#38434,#20590,.T.);
#49333=EDGE_CURVE('',#38432,#38434,#4225,.T.);
#49334=EDGE_CURVE('',#38435,#38436,#29035,.T.);
#49335=EDGE_CURVE('',#38435,#38431,#4226,.T.);
#49336=EDGE_CURVE('',#38436,#38432,#4227,.T.);
#49337=EDGE_CURVE('',#38437,#38438,#29036,.T.);
#49338=EDGE_CURVE('',#38437,#38435,#4228,.T.);
#49339=EDGE_CURVE('',#38438,#38436,#4229,.T.);
#49340=EDGE_CURVE('',#38439,#38440,#29037,.T.);
#49341=EDGE_CURVE('',#38439,#38437,#4230,.T.);
#49342=EDGE_CURVE('',#38440,#38438,#4231,.T.);
#49343=EDGE_CURVE('',#38441,#38442,#29038,.T.);
#49344=EDGE_CURVE('',#38441,#38439,#4232,.T.);
#49345=EDGE_CURVE('',#38442,#38440,#4233,.T.);
#49346=EDGE_CURVE('',#38443,#38444,#29039,.T.);
#49347=EDGE_CURVE('',#38443,#38441,#4234,.T.);
#49348=EDGE_CURVE('',#38444,#38442,#4235,.T.);
#49349=EDGE_CURVE('',#38445,#38446,#29040,.T.);
#49350=EDGE_CURVE('',#38445,#38443,#4236,.T.);
#49351=EDGE_CURVE('',#38446,#38444,#4237,.T.);
#49352=EDGE_CURVE('',#38447,#38448,#29041,.T.);
#49353=EDGE_CURVE('',#38447,#38445,#4238,.T.);
#49354=EDGE_CURVE('',#38448,#38446,#4239,.T.);
#49355=EDGE_CURVE('',#38449,#38450,#29042,.T.);
#49356=EDGE_CURVE('',#38449,#38447,#4240,.T.);
#49357=EDGE_CURVE('',#38450,#38448,#4241,.T.);
#49358=EDGE_CURVE('',#38451,#38452,#29043,.T.);
#49359=EDGE_CURVE('',#38451,#38449,#4242,.T.);
#49360=EDGE_CURVE('',#38452,#38450,#4243,.T.);
#49361=EDGE_CURVE('',#38453,#38454,#29044,.T.);
#49362=EDGE_CURVE('',#38453,#38451,#4244,.T.);
#49363=EDGE_CURVE('',#38454,#38452,#4245,.T.);
#49364=EDGE_CURVE('',#38455,#38456,#29045,.T.);
#49365=EDGE_CURVE('',#38455,#38453,#4246,.T.);
#49366=EDGE_CURVE('',#38456,#38454,#4247,.T.);
#49367=EDGE_CURVE('',#38457,#38458,#29046,.T.);
#49368=EDGE_CURVE('',#38457,#38455,#4248,.T.);
#49369=EDGE_CURVE('',#38458,#38456,#4249,.T.);
#49370=EDGE_CURVE('',#38459,#38460,#29047,.T.);
#49371=EDGE_CURVE('',#38459,#38457,#4250,.T.);
#49372=EDGE_CURVE('',#38460,#38458,#4251,.T.);
#49373=EDGE_CURVE('',#38461,#38462,#29048,.T.);
#49374=EDGE_CURVE('',#38463,#38461,#20591,.T.);
#49375=EDGE_CURVE('',#38463,#38459,#4252,.T.);
#49376=EDGE_CURVE('',#38462,#38460,#4253,.T.);
#49377=EDGE_CURVE('',#38464,#38465,#29049,.T.);
#49378=EDGE_CURVE('',#38466,#38464,#24674,.F.);
#49379=EDGE_CURVE('',#38466,#38467,#20592,.T.);
#49380=EDGE_CURVE('',#38467,#38465,#24675,.T.);
#49381=EDGE_CURVE('',#38468,#38469,#29050,.T.);
#49382=EDGE_CURVE('',#38464,#38468,#24676,.F.);
#49383=EDGE_CURVE('',#38465,#38469,#24677,.T.);
#49384=EDGE_CURVE('',#38470,#38471,#29051,.T.);
#49385=EDGE_CURVE('',#38468,#38470,#24678,.F.);
#49386=EDGE_CURVE('',#38469,#38471,#24679,.T.);
#49387=EDGE_CURVE('',#38472,#38473,#29052,.T.);
#49388=EDGE_CURVE('',#38470,#38472,#24680,.F.);
#49389=EDGE_CURVE('',#38471,#38473,#24681,.T.);
#49390=EDGE_CURVE('',#38474,#38475,#29053,.T.);
#49391=EDGE_CURVE('',#38472,#38474,#24682,.F.);
#49392=EDGE_CURVE('',#38473,#38475,#24683,.T.);
#49393=EDGE_CURVE('',#38476,#38477,#29054,.T.);
#49394=EDGE_CURVE('',#38474,#38476,#24684,.F.);
#49395=EDGE_CURVE('',#38475,#38477,#24685,.T.);
#49396=EDGE_CURVE('',#38478,#38479,#29055,.T.);
#49397=EDGE_CURVE('',#38476,#38478,#24686,.F.);
#49398=EDGE_CURVE('',#38477,#38479,#24687,.T.);
#49399=EDGE_CURVE('',#38480,#38481,#29056,.T.);
#49400=EDGE_CURVE('',#38478,#38480,#24688,.F.);
#49401=EDGE_CURVE('',#38479,#38481,#24689,.T.);
#49402=EDGE_CURVE('',#38482,#38483,#29057,.T.);
#49403=EDGE_CURVE('',#38480,#38482,#24690,.F.);
#49404=EDGE_CURVE('',#38481,#38483,#24691,.T.);
#49405=EDGE_CURVE('',#38484,#38485,#29058,.T.);
#49406=EDGE_CURVE('',#38482,#38484,#24692,.F.);
#49407=EDGE_CURVE('',#38483,#38485,#24693,.T.);
#49408=EDGE_CURVE('',#38486,#38487,#29059,.T.);
#49409=EDGE_CURVE('',#38484,#38486,#24694,.F.);
#49410=EDGE_CURVE('',#38485,#38487,#24695,.T.);
#49411=EDGE_CURVE('',#38488,#38489,#29060,.T.);
#49412=EDGE_CURVE('',#38486,#38488,#24696,.F.);
#49413=EDGE_CURVE('',#38487,#38489,#24697,.T.);
#49414=EDGE_CURVE('',#38490,#38491,#29061,.T.);
#49415=EDGE_CURVE('',#38488,#38490,#24698,.F.);
#49416=EDGE_CURVE('',#38489,#38491,#24699,.T.);
#49417=EDGE_CURVE('',#38492,#38493,#29062,.T.);
#49418=EDGE_CURVE('',#38490,#38492,#24700,.F.);
#49419=EDGE_CURVE('',#38491,#38493,#24701,.T.);
#49420=EDGE_CURVE('',#38461,#38494,#20593,.T.);
#49421=EDGE_CURVE('',#38494,#38467,#24702,.T.);
#49422=EDGE_CURVE('',#38466,#38495,#24703,.T.);
#49423=EDGE_CURVE('',#38495,#38496,#29063,.T.);
#49424=EDGE_CURVE('',#38496,#38496,#20594,.T.);
#49425=EDGE_CURVE('',#38495,#38463,#24704,.T.);
#49426=EDGE_CURVE('',#38493,#38497,#24705,.T.);
#49427=EDGE_CURVE('',#38498,#38497,#20595,.T.);
#49428=EDGE_CURVE('',#38492,#38498,#24706,.F.);
#49429=EDGE_CURVE('',#38499,#38500,#4254,.T.);
#49430=EDGE_CURVE('',#38499,#38500,#20596,.T.);
#49431=EDGE_CURVE('',#38501,#38501,#20597,.T.);
#49432=EDGE_CURVE('',#38501,#38502,#29064,.T.);
#49433=EDGE_CURVE('',#38502,#38502,#20598,.T.);
#49434=EDGE_CURVE('',#38502,#38503,#29065,.T.);
#49435=EDGE_CURVE('',#38503,#38504,#20599,.T.);
#49436=EDGE_CURVE('',#38498,#38504,#24707,.T.);
#49437=EDGE_CURVE('',#38505,#38497,#24708,.T.);
#49438=EDGE_CURVE('',#38505,#38503,#20600,.T.);
#49439=EDGE_CURVE('',#38500,#38506,#20601,.T.);
#49440=EDGE_CURVE('',#38506,#38507,#20602,.T.);
#49441=EDGE_CURVE('',#38507,#38508,#20603,.T.);
#49442=EDGE_CURVE('',#38508,#38509,#20604,.T.);
#49443=EDGE_CURVE('',#38509,#38499,#20605,.T.);
#49444=EDGE_CURVE('',#38504,#38433,#24709,.T.);
#49445=EDGE_CURVE('',#38434,#38505,#24710,.T.);
#49446=EDGE_CURVE('',#38507,#38508,#4255,.T.);
#49447=EDGE_CURVE('',#38506,#38507,#4256,.T.);
#49448=EDGE_CURVE('',#38500,#38506,#4257,.T.);
#49449=EDGE_CURVE('',#38509,#38499,#4258,.T.);
#49450=EDGE_CURVE('',#38508,#38509,#4259,.T.);
#49451=EDGE_CURVE('',#38510,#38511,#29066,.T.);
#49452=EDGE_CURVE('',#38511,#38512,#29067,.T.);
#49453=EDGE_CURVE('',#38512,#38513,#29068,.T.);
#49454=EDGE_CURVE('',#38513,#38514,#29069,.T.);
#49455=EDGE_CURVE('',#38514,#38515,#29070,.T.);
#49456=EDGE_CURVE('',#38515,#38510,#29071,.T.);
#49457=EDGE_CURVE('',#38512,#38507,#29072,.T.);
#49458=EDGE_CURVE('',#38511,#38508,#29073,.T.);
#49459=EDGE_CURVE('',#38513,#38506,#29074,.T.);
#49460=EDGE_CURVE('',#38514,#38500,#29075,.T.);
#49461=EDGE_CURVE('',#38515,#38499,#29076,.T.);
#49462=EDGE_CURVE('',#38510,#38509,#29077,.T.);
#49463=EDGE_CURVE('',#38494,#38462,#4260,.T.);
#69656=ORIENTED_EDGE('',*,*,#49330,.F.);
#69657=ORIENTED_EDGE('',*,*,#49331,.T.);
#69658=ORIENTED_EDGE('',*,*,#49332,.T.);
#69659=ORIENTED_EDGE('',*,*,#49333,.F.);
#69660=ORIENTED_EDGE('',*,*,#49334,.F.);
#69661=ORIENTED_EDGE('',*,*,#49335,.T.);
#69662=ORIENTED_EDGE('',*,*,#49330,.T.);
#69663=ORIENTED_EDGE('',*,*,#49336,.F.);
#69664=ORIENTED_EDGE('',*,*,#49337,.F.);
#69665=ORIENTED_EDGE('',*,*,#49338,.T.);
#69666=ORIENTED_EDGE('',*,*,#49334,.T.);
#69667=ORIENTED_EDGE('',*,*,#49339,.F.);
#69668=ORIENTED_EDGE('',*,*,#49340,.F.);
#69669=ORIENTED_EDGE('',*,*,#49341,.T.);
#69670=ORIENTED_EDGE('',*,*,#49337,.T.);
#69671=ORIENTED_EDGE('',*,*,#49342,.F.);
#69672=ORIENTED_EDGE('',*,*,#49343,.F.);
#69673=ORIENTED_EDGE('',*,*,#49344,.T.);
#69674=ORIENTED_EDGE('',*,*,#49340,.T.);
#69675=ORIENTED_EDGE('',*,*,#49345,.F.);
#69676=ORIENTED_EDGE('',*,*,#49346,.F.);
#69677=ORIENTED_EDGE('',*,*,#49347,.T.);
#69678=ORIENTED_EDGE('',*,*,#49343,.T.);
#69679=ORIENTED_EDGE('',*,*,#49348,.F.);
#69680=ORIENTED_EDGE('',*,*,#49349,.F.);
#69681=ORIENTED_EDGE('',*,*,#49350,.T.);
#69682=ORIENTED_EDGE('',*,*,#49346,.T.);
#69683=ORIENTED_EDGE('',*,*,#49351,.F.);
#69684=ORIENTED_EDGE('',*,*,#49352,.F.);
#69685=ORIENTED_EDGE('',*,*,#49353,.T.);
#69686=ORIENTED_EDGE('',*,*,#49349,.T.);
#69687=ORIENTED_EDGE('',*,*,#49354,.F.);
#69688=ORIENTED_EDGE('',*,*,#49355,.F.);
#69689=ORIENTED_EDGE('',*,*,#49356,.T.);
#69690=ORIENTED_EDGE('',*,*,#49352,.T.);
#69691=ORIENTED_EDGE('',*,*,#49357,.F.);
#69692=ORIENTED_EDGE('',*,*,#49358,.F.);
#69693=ORIENTED_EDGE('',*,*,#49359,.T.);
#69694=ORIENTED_EDGE('',*,*,#49355,.T.);
#69695=ORIENTED_EDGE('',*,*,#49360,.F.);
#69696=ORIENTED_EDGE('',*,*,#49361,.F.);
#69697=ORIENTED_EDGE('',*,*,#49362,.T.);
#69698=ORIENTED_EDGE('',*,*,#49358,.T.);
#69699=ORIENTED_EDGE('',*,*,#49363,.F.);
#69700=ORIENTED_EDGE('',*,*,#49364,.F.);
#69701=ORIENTED_EDGE('',*,*,#49365,.T.);
#69702=ORIENTED_EDGE('',*,*,#49361,.T.);
#69703=ORIENTED_EDGE('',*,*,#49366,.F.);
#69704=ORIENTED_EDGE('',*,*,#49367,.F.);
#69705=ORIENTED_EDGE('',*,*,#49368,.T.);
#69706=ORIENTED_EDGE('',*,*,#49364,.T.);
#69707=ORIENTED_EDGE('',*,*,#49369,.F.);
#69708=ORIENTED_EDGE('',*,*,#49370,.F.);
#69709=ORIENTED_EDGE('',*,*,#49371,.T.);
#69710=ORIENTED_EDGE('',*,*,#49367,.T.);
#69711=ORIENTED_EDGE('',*,*,#49372,.F.);
#69712=ORIENTED_EDGE('',*,*,#49373,.F.);
#69713=ORIENTED_EDGE('',*,*,#49374,.F.);
#69714=ORIENTED_EDGE('',*,*,#49375,.T.);
#69715=ORIENTED_EDGE('',*,*,#49370,.T.);
#69716=ORIENTED_EDGE('',*,*,#49376,.F.);
#69717=ORIENTED_EDGE('',*,*,#49377,.F.);
#69718=ORIENTED_EDGE('',*,*,#49378,.F.);
#69719=ORIENTED_EDGE('',*,*,#49379,.T.);
#69720=ORIENTED_EDGE('',*,*,#49380,.T.);
#69721=ORIENTED_EDGE('',*,*,#49381,.F.);
#69722=ORIENTED_EDGE('',*,*,#49382,.F.);
#69723=ORIENTED_EDGE('',*,*,#49377,.T.);
#69724=ORIENTED_EDGE('',*,*,#49383,.T.);
#69725=ORIENTED_EDGE('',*,*,#49384,.F.);
#69726=ORIENTED_EDGE('',*,*,#49385,.F.);
#69727=ORIENTED_EDGE('',*,*,#49381,.T.);
#69728=ORIENTED_EDGE('',*,*,#49386,.T.);
#69729=ORIENTED_EDGE('',*,*,#49387,.F.);
#69730=ORIENTED_EDGE('',*,*,#49388,.F.);
#69731=ORIENTED_EDGE('',*,*,#49384,.T.);
#69732=ORIENTED_EDGE('',*,*,#49389,.T.);
#69733=ORIENTED_EDGE('',*,*,#49390,.F.);
#69734=ORIENTED_EDGE('',*,*,#49391,.F.);
#69735=ORIENTED_EDGE('',*,*,#49387,.T.);
#69736=ORIENTED_EDGE('',*,*,#49392,.T.);
#69737=ORIENTED_EDGE('',*,*,#49393,.F.);
#69738=ORIENTED_EDGE('',*,*,#49394,.F.);
#69739=ORIENTED_EDGE('',*,*,#49390,.T.);
#69740=ORIENTED_EDGE('',*,*,#49395,.T.);
#69741=ORIENTED_EDGE('',*,*,#49396,.F.);
#69742=ORIENTED_EDGE('',*,*,#49397,.F.);
#69743=ORIENTED_EDGE('',*,*,#49393,.T.);
#69744=ORIENTED_EDGE('',*,*,#49398,.T.);
#69745=ORIENTED_EDGE('',*,*,#49399,.F.);
#69746=ORIENTED_EDGE('',*,*,#49400,.F.);
#69747=ORIENTED_EDGE('',*,*,#49396,.T.);
#69748=ORIENTED_EDGE('',*,*,#49401,.T.);
#69749=ORIENTED_EDGE('',*,*,#49402,.F.);
#69750=ORIENTED_EDGE('',*,*,#49403,.F.);
#69751=ORIENTED_EDGE('',*,*,#49399,.T.);
#69752=ORIENTED_EDGE('',*,*,#49404,.T.);
#69753=ORIENTED_EDGE('',*,*,#49405,.F.);
#69754=ORIENTED_EDGE('',*,*,#49406,.F.);
#69755=ORIENTED_EDGE('',*,*,#49402,.T.);
#69756=ORIENTED_EDGE('',*,*,#49407,.T.);
#69757=ORIENTED_EDGE('',*,*,#49408,.F.);
#69758=ORIENTED_EDGE('',*,*,#49409,.F.);
#69759=ORIENTED_EDGE('',*,*,#49405,.T.);
#69760=ORIENTED_EDGE('',*,*,#49410,.T.);
#69761=ORIENTED_EDGE('',*,*,#49411,.F.);
#69762=ORIENTED_EDGE('',*,*,#49412,.F.);
#69763=ORIENTED_EDGE('',*,*,#49408,.T.);
#69764=ORIENTED_EDGE('',*,*,#49413,.T.);
#69765=ORIENTED_EDGE('',*,*,#49414,.F.);
#69766=ORIENTED_EDGE('',*,*,#49415,.F.);
#69767=ORIENTED_EDGE('',*,*,#49411,.T.);
#69768=ORIENTED_EDGE('',*,*,#49416,.T.);
#69769=ORIENTED_EDGE('',*,*,#49417,.F.);
#69770=ORIENTED_EDGE('',*,*,#49418,.F.);
#69771=ORIENTED_EDGE('',*,*,#49414,.T.);
#69772=ORIENTED_EDGE('',*,*,#49419,.T.);
#69773=ORIENTED_EDGE('',*,*,#49374,.T.);
#69774=ORIENTED_EDGE('',*,*,#49420,.T.);
#69775=ORIENTED_EDGE('',*,*,#49421,.T.);
#69776=ORIENTED_EDGE('',*,*,#49379,.F.);
#69777=ORIENTED_EDGE('',*,*,#49422,.T.);
#69778=ORIENTED_EDGE('',*,*,#49423,.T.);
#69779=ORIENTED_EDGE('',*,*,#49424,.F.);
#69780=ORIENTED_EDGE('',*,*,#49423,.F.);
#69781=ORIENTED_EDGE('',*,*,#49425,.T.);
#69782=ORIENTED_EDGE('',*,*,#49417,.T.);
#69783=ORIENTED_EDGE('',*,*,#49426,.T.);
#69784=ORIENTED_EDGE('',*,*,#49427,.F.);
#69785=ORIENTED_EDGE('',*,*,#49428,.F.);
#69786=ORIENTED_EDGE('',*,*,#49429,.T.);
#69787=ORIENTED_EDGE('',*,*,#49430,.F.);
#69788=ORIENTED_EDGE('',*,*,#49431,.F.);
#69789=ORIENTED_EDGE('',*,*,#49432,.T.);
#69790=ORIENTED_EDGE('',*,*,#49433,.T.);
#69791=ORIENTED_EDGE('',*,*,#49432,.F.);
#69792=ORIENTED_EDGE('',*,*,#49433,.F.);
#69793=ORIENTED_EDGE('',*,*,#49434,.T.);
#69794=ORIENTED_EDGE('',*,*,#49435,.T.);
#69795=ORIENTED_EDGE('',*,*,#49436,.F.);
#69796=ORIENTED_EDGE('',*,*,#49427,.T.);
#69797=ORIENTED_EDGE('',*,*,#49437,.F.);
#69798=ORIENTED_EDGE('',*,*,#49438,.T.);
#69799=ORIENTED_EDGE('',*,*,#49434,.F.);
#69800=ORIENTED_EDGE('',*,*,#49431,.T.);
#69801=ORIENTED_EDGE('',*,*,#49439,.T.);
#69802=ORIENTED_EDGE('',*,*,#49440,.T.);
#69803=ORIENTED_EDGE('',*,*,#49441,.T.);
#69804=ORIENTED_EDGE('',*,*,#49442,.T.);
#69805=ORIENTED_EDGE('',*,*,#49443,.T.);
#69806=ORIENTED_EDGE('',*,*,#49430,.T.);
#69807=ORIENTED_EDGE('',*,*,#49444,.F.);
#69808=ORIENTED_EDGE('',*,*,#49435,.F.);
#69809=ORIENTED_EDGE('',*,*,#49438,.F.);
#69810=ORIENTED_EDGE('',*,*,#49445,.F.);
#69811=ORIENTED_EDGE('',*,*,#49332,.F.);
#69812=ORIENTED_EDGE('',*,*,#49446,.T.);
#69813=ORIENTED_EDGE('',*,*,#49441,.F.);
#69814=ORIENTED_EDGE('',*,*,#49447,.T.);
#69815=ORIENTED_EDGE('',*,*,#49440,.F.);
#69816=ORIENTED_EDGE('',*,*,#49448,.T.);
#69817=ORIENTED_EDGE('',*,*,#49439,.F.);
#69818=ORIENTED_EDGE('',*,*,#49449,.T.);
#69819=ORIENTED_EDGE('',*,*,#49443,.F.);
#69820=ORIENTED_EDGE('',*,*,#49450,.T.);
#69821=ORIENTED_EDGE('',*,*,#49442,.F.);
#69822=ORIENTED_EDGE('',*,*,#49451,.T.);
#69823=ORIENTED_EDGE('',*,*,#49452,.T.);
#69824=ORIENTED_EDGE('',*,*,#49453,.T.);
#69825=ORIENTED_EDGE('',*,*,#49454,.T.);
#69826=ORIENTED_EDGE('',*,*,#49455,.T.);
#69827=ORIENTED_EDGE('',*,*,#49456,.T.);
#69828=ORIENTED_EDGE('',*,*,#49446,.F.);
#69829=ORIENTED_EDGE('',*,*,#49457,.F.);
#69830=ORIENTED_EDGE('',*,*,#49452,.F.);
#69831=ORIENTED_EDGE('',*,*,#49458,.T.);
#69832=ORIENTED_EDGE('',*,*,#49447,.F.);
#69833=ORIENTED_EDGE('',*,*,#49459,.F.);
#69834=ORIENTED_EDGE('',*,*,#49453,.F.);
#69835=ORIENTED_EDGE('',*,*,#49457,.T.);
#69836=ORIENTED_EDGE('',*,*,#49448,.F.);
#69837=ORIENTED_EDGE('',*,*,#49460,.F.);
#69838=ORIENTED_EDGE('',*,*,#49454,.F.);
#69839=ORIENTED_EDGE('',*,*,#49459,.T.);
#69840=ORIENTED_EDGE('',*,*,#49429,.F.);
#69841=ORIENTED_EDGE('',*,*,#49461,.F.);
#69842=ORIENTED_EDGE('',*,*,#49455,.F.);
#69843=ORIENTED_EDGE('',*,*,#49460,.T.);
#69844=ORIENTED_EDGE('',*,*,#49449,.F.);
#69845=ORIENTED_EDGE('',*,*,#49462,.F.);
#69846=ORIENTED_EDGE('',*,*,#49456,.F.);
#69847=ORIENTED_EDGE('',*,*,#49461,.T.);
#69848=ORIENTED_EDGE('',*,*,#49450,.F.);
#69849=ORIENTED_EDGE('',*,*,#49458,.F.);
#69850=ORIENTED_EDGE('',*,*,#49451,.F.);
#69851=ORIENTED_EDGE('',*,*,#49462,.T.);
#69852=ORIENTED_EDGE('',*,*,#49424,.T.);
#69853=ORIENTED_EDGE('',*,*,#49378,.T.);
#69854=ORIENTED_EDGE('',*,*,#49382,.T.);
#69855=ORIENTED_EDGE('',*,*,#49385,.T.);
#69856=ORIENTED_EDGE('',*,*,#49388,.T.);
#69857=ORIENTED_EDGE('',*,*,#49391,.T.);
#69858=ORIENTED_EDGE('',*,*,#49394,.T.);
#69859=ORIENTED_EDGE('',*,*,#49397,.T.);
#69860=ORIENTED_EDGE('',*,*,#49400,.T.);
#69861=ORIENTED_EDGE('',*,*,#49403,.T.);
#69862=ORIENTED_EDGE('',*,*,#49406,.T.);
#69863=ORIENTED_EDGE('',*,*,#49409,.T.);
#69864=ORIENTED_EDGE('',*,*,#49412,.T.);
#69865=ORIENTED_EDGE('',*,*,#49415,.T.);
#69866=ORIENTED_EDGE('',*,*,#49418,.T.);
#69867=ORIENTED_EDGE('',*,*,#49428,.T.);
#69868=ORIENTED_EDGE('',*,*,#49436,.T.);
#69869=ORIENTED_EDGE('',*,*,#49444,.T.);
#69870=ORIENTED_EDGE('',*,*,#49331,.F.);
#69871=ORIENTED_EDGE('',*,*,#49335,.F.);
#69872=ORIENTED_EDGE('',*,*,#49338,.F.);
#69873=ORIENTED_EDGE('',*,*,#49341,.F.);
#69874=ORIENTED_EDGE('',*,*,#49344,.F.);
#69875=ORIENTED_EDGE('',*,*,#49347,.F.);
#69876=ORIENTED_EDGE('',*,*,#49350,.F.);
#69877=ORIENTED_EDGE('',*,*,#49353,.F.);
#69878=ORIENTED_EDGE('',*,*,#49356,.F.);
#69879=ORIENTED_EDGE('',*,*,#49359,.F.);
#69880=ORIENTED_EDGE('',*,*,#49362,.F.);
#69881=ORIENTED_EDGE('',*,*,#49365,.F.);
#69882=ORIENTED_EDGE('',*,*,#49368,.F.);
#69883=ORIENTED_EDGE('',*,*,#49371,.F.);
#69884=ORIENTED_EDGE('',*,*,#49375,.F.);
#69885=ORIENTED_EDGE('',*,*,#49425,.F.);
#69886=ORIENTED_EDGE('',*,*,#49422,.F.);
#69887=ORIENTED_EDGE('',*,*,#49373,.T.);
#69888=ORIENTED_EDGE('',*,*,#49463,.F.);
#69889=ORIENTED_EDGE('',*,*,#49420,.F.);
#69890=ORIENTED_EDGE('',*,*,#49445,.T.);
#69891=ORIENTED_EDGE('',*,*,#49437,.T.);
#69892=ORIENTED_EDGE('',*,*,#49426,.F.);
#69893=ORIENTED_EDGE('',*,*,#49419,.F.);
#69894=ORIENTED_EDGE('',*,*,#49416,.F.);
#69895=ORIENTED_EDGE('',*,*,#49413,.F.);
#69896=ORIENTED_EDGE('',*,*,#49410,.F.);
#69897=ORIENTED_EDGE('',*,*,#49407,.F.);
#69898=ORIENTED_EDGE('',*,*,#49404,.F.);
#69899=ORIENTED_EDGE('',*,*,#49401,.F.);
#69900=ORIENTED_EDGE('',*,*,#49398,.F.);
#69901=ORIENTED_EDGE('',*,*,#49395,.F.);
#69902=ORIENTED_EDGE('',*,*,#49392,.F.);
#69903=ORIENTED_EDGE('',*,*,#49389,.F.);
#69904=ORIENTED_EDGE('',*,*,#49386,.F.);
#69905=ORIENTED_EDGE('',*,*,#49383,.F.);
#69906=ORIENTED_EDGE('',*,*,#49380,.F.);
#69907=ORIENTED_EDGE('',*,*,#49421,.F.);
#69908=ORIENTED_EDGE('',*,*,#49463,.T.);
#69909=ORIENTED_EDGE('',*,*,#49376,.T.);
#69910=ORIENTED_EDGE('',*,*,#49372,.T.);
#69911=ORIENTED_EDGE('',*,*,#49369,.T.);
#69912=ORIENTED_EDGE('',*,*,#49366,.T.);
#69913=ORIENTED_EDGE('',*,*,#49363,.T.);
#69914=ORIENTED_EDGE('',*,*,#49360,.T.);
#69915=ORIENTED_EDGE('',*,*,#49357,.T.);
#69916=ORIENTED_EDGE('',*,*,#49354,.T.);
#69917=ORIENTED_EDGE('',*,*,#49351,.T.);
#69918=ORIENTED_EDGE('',*,*,#49348,.T.);
#69919=ORIENTED_EDGE('',*,*,#49345,.T.);
#69920=ORIENTED_EDGE('',*,*,#49342,.T.);
#69921=ORIENTED_EDGE('',*,*,#49339,.T.);
#69922=ORIENTED_EDGE('',*,*,#49336,.T.);
#69923=ORIENTED_EDGE('',*,*,#49333,.T.);
#87965=CYLINDRICAL_SURFACE('',#99319,0.957716426222737);
#87966=CYLINDRICAL_SURFACE('',#99321,0.957716426222737);
#87967=CYLINDRICAL_SURFACE('',#99322,0.957716426222737);
#87968=CYLINDRICAL_SURFACE('',#99323,0.957716426222737);
#87969=CYLINDRICAL_SURFACE('',#99324,0.957716426222737);
#87970=CYLINDRICAL_SURFACE('',#99325,0.957716426222737);
#87971=CYLINDRICAL_SURFACE('',#99326,0.957716426222737);
#87972=CYLINDRICAL_SURFACE('',#99327,0.957716426222737);
#87973=CYLINDRICAL_SURFACE('',#99328,0.957716426222737);
#87974=CYLINDRICAL_SURFACE('',#99329,0.957716426222737);
#87975=CYLINDRICAL_SURFACE('',#99330,0.957716426222737);
#87976=CYLINDRICAL_SURFACE('',#99331,0.957716426222737);
#87977=CYLINDRICAL_SURFACE('',#99332,0.957716426222737);
#87978=CYLINDRICAL_SURFACE('',#99333,0.957716426222737);
#87979=CYLINDRICAL_SURFACE('',#99334,0.957716426222737);
#87980=CYLINDRICAL_SURFACE('',#99336,1.25000000000001);
#87981=CYLINDRICAL_SURFACE('',#99338,1.25000000000001);
#87982=CYLINDRICAL_SURFACE('',#99339,1.25000000000001);
#87983=CYLINDRICAL_SURFACE('',#99340,1.25000000000001);
#87984=CYLINDRICAL_SURFACE('',#99341,1.25000000000001);
#87985=CYLINDRICAL_SURFACE('',#99342,1.25000000000001);
#87986=CYLINDRICAL_SURFACE('',#99343,1.25000000000001);
#87987=CYLINDRICAL_SURFACE('',#99344,1.25000000000001);
#87988=CYLINDRICAL_SURFACE('',#99345,1.25000000000001);
#87989=CYLINDRICAL_SURFACE('',#99346,1.25000000000001);
#87990=CYLINDRICAL_SURFACE('',#99347,1.25000000000001);
#87991=CYLINDRICAL_SURFACE('',#99348,1.25000000000001);
#87992=CYLINDRICAL_SURFACE('',#99349,1.25000000000001);
#87993=CYLINDRICAL_SURFACE('',#99350,1.25000000000001);
#87994=CYLINDRICAL_SURFACE('',#99354,1.25000000000001);
#87995=CYLINDRICAL_SURFACE('',#99358,2.5);
#87996=CYLINDRICAL_SURFACE('',#99384,0.957716426222737);
#90963=ADVANCED_FACE('',(#8499),#87965,.T.);
#90964=ADVANCED_FACE('',(#8500),#87966,.T.);
#90965=ADVANCED_FACE('',(#8501),#87967,.T.);
#90966=ADVANCED_FACE('',(#8502),#87968,.T.);
#90967=ADVANCED_FACE('',(#8503),#87969,.T.);
#90968=ADVANCED_FACE('',(#8504),#87970,.T.);
#90969=ADVANCED_FACE('',(#8505),#87971,.T.);
#90970=ADVANCED_FACE('',(#8506),#87972,.T.);
#90971=ADVANCED_FACE('',(#8507),#87973,.T.);
#90972=ADVANCED_FACE('',(#8508),#87974,.T.);
#90973=ADVANCED_FACE('',(#8509),#87975,.T.);
#90974=ADVANCED_FACE('',(#8510),#87976,.T.);
#90975=ADVANCED_FACE('',(#8511),#87977,.T.);
#90976=ADVANCED_FACE('',(#8512),#87978,.T.);
#90977=ADVANCED_FACE('',(#8513),#87979,.T.);
#90978=ADVANCED_FACE('',(#8514),#87980,.T.);
#90979=ADVANCED_FACE('',(#8515),#87981,.T.);
#90980=ADVANCED_FACE('',(#8516),#87982,.T.);
#90981=ADVANCED_FACE('',(#8517),#87983,.T.);
#90982=ADVANCED_FACE('',(#8518),#87984,.T.);
#90983=ADVANCED_FACE('',(#8519),#87985,.T.);
#90984=ADVANCED_FACE('',(#8520),#87986,.T.);
#90985=ADVANCED_FACE('',(#8521),#87987,.T.);
#90986=ADVANCED_FACE('',(#8522),#87988,.T.);
#90987=ADVANCED_FACE('',(#8523),#87989,.T.);
#90988=ADVANCED_FACE('',(#8524),#87990,.T.);
#90989=ADVANCED_FACE('',(#8525),#87991,.T.);
#90990=ADVANCED_FACE('',(#8526),#87992,.T.);
#90991=ADVANCED_FACE('',(#8527),#87993,.T.);
#90992=ADVANCED_FACE('',(#8528),#4895,.T.);
#90993=ADVANCED_FACE('',(#8529),#87994,.T.);
#90994=ADVANCED_FACE('',(#8530),#4896,.F.);
#90995=ADVANCED_FACE('',(#8531),#87995,.T.);
#90996=ADVANCED_FACE('',(#8532),#4897,.T.);
#90997=ADVANCED_FACE('',(#8533,#5225),#5716,.F.);
#90998=ADVANCED_FACE('',(#8534),#5717,.T.);
#90999=ADVANCED_FACE('',(#8535),#4898,.F.);
#91000=ADVANCED_FACE('',(#8536),#4899,.F.);
#91001=ADVANCED_FACE('',(#8537),#4900,.F.);
#91002=ADVANCED_FACE('',(#8538),#4901,.F.);
#91003=ADVANCED_FACE('',(#8539),#4902,.F.);
#91004=ADVANCED_FACE('',(#8540),#5718,.T.);
#91005=ADVANCED_FACE('',(#8541),#5719,.F.);
#91006=ADVANCED_FACE('',(#8542),#5720,.F.);
#91007=ADVANCED_FACE('',(#8543),#5721,.F.);
#91008=ADVANCED_FACE('',(#8544),#5722,.F.);
#91009=ADVANCED_FACE('',(#8545),#5723,.F.);
#91010=ADVANCED_FACE('',(#8546),#5724,.F.);
#91011=ADVANCED_FACE('',(#8547),#5725,.F.);
#91012=ADVANCED_FACE('',(#8548),#2317,.T.);
#91013=ADVANCED_FACE('',(#8549),#87996,.T.);
#91014=ADVANCED_FACE('',(#8550),#2318,.T.);
#94664=CLOSED_SHELL('',(#90963,#90964,#90965,#90966,#90967,#90968,#90969,
#90970,#90971,#90972,#90973,#90974,#90975,#90976,#90977,#90978,#90979,#90980,
#90981,#90982,#90983,#90984,#90985,#90986,#90987,#90988,#90989,#90990,#90991,
#90992,#90993,#90994,#90995,#90996,#90997,#90998,#90999,#91000,#91001,#91002,
#91003,#91004,#91005,#91006,#91007,#91008,#91009,#91010,#91011,#91012,#91013,
#91014));
#99318=AXIS2_PLACEMENT_3D('',#368987,#116390,#116391);
#99319=AXIS2_PLACEMENT_3D('',#368988,#116392,#116393);
#99320=AXIS2_PLACEMENT_3D('',#369001,#116395,#116396);
#99321=AXIS2_PLACEMENT_3D('',#369007,#116397,#116398);
#99322=AXIS2_PLACEMENT_3D('',#369037,#116400,#116401);
#99323=AXIS2_PLACEMENT_3D('',#369067,#116403,#116404);
#99324=AXIS2_PLACEMENT_3D('',#369097,#116406,#116407);
#99325=AXIS2_PLACEMENT_3D('',#369127,#116409,#116410);
#99326=AXIS2_PLACEMENT_3D('',#369157,#116412,#116413);
#99327=AXIS2_PLACEMENT_3D('',#369187,#116415,#116416);
#99328=AXIS2_PLACEMENT_3D('',#369217,#116418,#116419);
#99329=AXIS2_PLACEMENT_3D('',#369247,#116421,#116422);
#99330=AXIS2_PLACEMENT_3D('',#369277,#116424,#116425);
#99331=AXIS2_PLACEMENT_3D('',#369307,#116427,#116428);
#99332=AXIS2_PLACEMENT_3D('',#369337,#116430,#116431);
#99333=AXIS2_PLACEMENT_3D('',#369367,#116433,#116434);
#99334=AXIS2_PLACEMENT_3D('',#369397,#116436,#116437);
#99335=AXIS2_PLACEMENT_3D('',#369402,#116439,#116440);
#99336=AXIS2_PLACEMENT_3D('',#369429,#116441,#116442);
#99337=AXIS2_PLACEMENT_3D('',#369451,#116444,#116445);
#99338=AXIS2_PLACEMENT_3D('',#369464,#116446,#116447);
#99339=AXIS2_PLACEMENT_3D('',#369540,#116449,#116450);
#99340=AXIS2_PLACEMENT_3D('',#369616,#116452,#116453);
#99341=AXIS2_PLACEMENT_3D('',#369692,#116455,#116456);
#99342=AXIS2_PLACEMENT_3D('',#369768,#116458,#116459);
#99343=AXIS2_PLACEMENT_3D('',#369846,#116461,#116462);
#99344=AXIS2_PLACEMENT_3D('',#369924,#116464,#116465);
#99345=AXIS2_PLACEMENT_3D('',#370000,#116467,#116468);
#99346=AXIS2_PLACEMENT_3D('',#370076,#116470,#116471);
#99347=AXIS2_PLACEMENT_3D('',#370152,#116473,#116474);
#99348=AXIS2_PLACEMENT_3D('',#370228,#116476,#116477);
#99349=AXIS2_PLACEMENT_3D('',#370304,#116479,#116480);
#99350=AXIS2_PLACEMENT_3D('',#370382,#116482,#116483);
#99351=AXIS2_PLACEMENT_3D('',#370460,#116485,#116486);
#99352=AXIS2_PLACEMENT_3D('',#370462,#116487,#116488);
#99353=AXIS2_PLACEMENT_3D('',#370502,#116490,#116491);
#99354=AXIS2_PLACEMENT_3D('',#370521,#116492,#116493);
#99355=AXIS2_PLACEMENT_3D('',#370554,#116494,#116495);
#99356=AXIS2_PLACEMENT_3D('',#370581,#116496,#116497);
#99357=AXIS2_PLACEMENT_3D('',#370587,#116498,#116499);
#99358=AXIS2_PLACEMENT_3D('',#370588,#116500,#116501);
#99359=AXIS2_PLACEMENT_3D('',#370590,#116502,#116503);
#99360=AXIS2_PLACEMENT_3D('',#370593,#116505,#116506);
#99361=AXIS2_PLACEMENT_3D('',#370594,#116507,#116508);
#99362=AXIS2_PLACEMENT_3D('',#370598,#116510,#116511);
#99363=AXIS2_PLACEMENT_3D('',#370661,#116512,#116513);
#99364=AXIS2_PLACEMENT_3D('',#370662,#116514,#116515);
#99365=AXIS2_PLACEMENT_3D('',#370664,#116516,#116517);
#99366=AXIS2_PLACEMENT_3D('',#370666,#116518,#116519);
#99367=AXIS2_PLACEMENT_3D('',#370668,#116520,#116521);
#99368=AXIS2_PLACEMENT_3D('',#370670,#116522,#116523);
#99369=AXIS2_PLACEMENT_3D('',#370671,#116524,#116525);
#99370=AXIS2_PLACEMENT_3D('',#370672,#116526,#116527);
#99371=AXIS2_PLACEMENT_3D('',#370693,#116528,#116529);
#99372=AXIS2_PLACEMENT_3D('',#370697,#116530,#116531);
#99373=AXIS2_PLACEMENT_3D('',#370701,#116532,#116533);
#99374=AXIS2_PLACEMENT_3D('',#370705,#116534,#116535);
#99375=AXIS2_PLACEMENT_3D('',#370709,#116536,#116537);
#99376=AXIS2_PLACEMENT_3D('',#370713,#116538,#116539);
#99377=AXIS2_PLACEMENT_3D('',#370726,#116546,#116547);
#99378=AXIS2_PLACEMENT_3D('',#370729,#116550,#116551);
#99379=AXIS2_PLACEMENT_3D('',#370731,#116553,#116554);
#99380=AXIS2_PLACEMENT_3D('',#370733,#116556,#116557);
#99381=AXIS2_PLACEMENT_3D('',#370735,#116559,#116560);
#99382=AXIS2_PLACEMENT_3D('',#370737,#116562,#116563);
#99383=AXIS2_PLACEMENT_3D('',#370738,#116564,#116565);
#99384=AXIS2_PLACEMENT_3D('',#371173,#116566,#116567);
#116390=DIRECTION('axis',(0.,0.,1.));
#116391=DIRECTION('refdir',(1.,0.,0.));
#116392=DIRECTION('center_axis',(-1.02434006807916E-22,-1.4843197546388E-38,
-1.));
#116393=DIRECTION('ref_axis',(-1.4490497842403E-16,1.,0.));
#116394=DIRECTION('',(1.02434006807916E-22,1.4843197546388E-38,1.));
#116395=DIRECTION('center_axis',(0.,-6.8448976313476E-17,-1.));
#116396=DIRECTION('ref_axis',(-1.4490497842403E-16,1.,0.));
#116397=DIRECTION('center_axis',(-1.02434006807916E-22,-1.4843197546388E-38,
-1.));
#116398=DIRECTION('ref_axis',(-1.4490497842403E-16,1.,0.));
#116399=DIRECTION('',(1.02434006807916E-22,1.4843197546388E-38,1.));
#116400=DIRECTION('center_axis',(-1.02434006807916E-22,-1.4843197546388E-38,
-1.));
#116401=DIRECTION('ref_axis',(-1.4490497842403E-16,1.,0.));
#116402=DIRECTION('',(1.02434006807916E-22,1.4843197546388E-38,1.));
#116403=DIRECTION('center_axis',(-1.02434006807916E-22,-1.4843197546388E-38,
-1.));
#116404=DIRECTION('ref_axis',(-1.4490497842403E-16,1.,0.));
#116405=DIRECTION('',(1.02434006807916E-22,1.4843197546388E-38,1.));
#116406=DIRECTION('center_axis',(-1.02434006807916E-22,-1.4843197546388E-38,
-1.));
#116407=DIRECTION('ref_axis',(-1.4490497842403E-16,1.,0.));
#116408=DIRECTION('',(1.02434006807916E-22,1.4843197546388E-38,1.));
#116409=DIRECTION('center_axis',(-1.02434006807916E-22,-1.4843197546388E-38,
-1.));
#116410=DIRECTION('ref_axis',(-1.4490497842403E-16,1.,0.));
#116411=DIRECTION('',(1.02434006807916E-22,1.4843197546388E-38,1.));
#116412=DIRECTION('center_axis',(-1.02434006807916E-22,-1.4843197546388E-38,
-1.));
#116413=DIRECTION('ref_axis',(-1.4490497842403E-16,1.,0.));
#116414=DIRECTION('',(1.02434006807916E-22,1.4843197546388E-38,1.));
#116415=DIRECTION('center_axis',(-1.02434006807916E-22,-1.4843197546388E-38,
-1.));
#116416=DIRECTION('ref_axis',(-1.4490497842403E-16,1.,0.));
#116417=DIRECTION('',(1.02434006807916E-22,1.4843197546388E-38,1.));
#116418=DIRECTION('center_axis',(-1.02434006807916E-22,-1.4843197546388E-38,
-1.));
#116419=DIRECTION('ref_axis',(-1.4490497842403E-16,1.,0.));
#116420=DIRECTION('',(1.02434006807916E-22,1.4843197546388E-38,1.));
#116421=DIRECTION('center_axis',(-1.02434006807916E-22,-1.4843197546388E-38,
-1.));
#116422=DIRECTION('ref_axis',(-1.4490497842403E-16,1.,0.));
#116423=DIRECTION('',(1.02434006807916E-22,1.4843197546388E-38,1.));
#116424=DIRECTION('center_axis',(-1.02434006807916E-22,-1.4843197546388E-38,
-1.));
#116425=DIRECTION('ref_axis',(-1.4490497842403E-16,1.,0.));
#116426=DIRECTION('',(1.02434006807916E-22,1.4843197546388E-38,1.));
#116427=DIRECTION('center_axis',(-1.02434006807916E-22,-1.4843197546388E-38,
-1.));
#116428=DIRECTION('ref_axis',(-1.4490497842403E-16,1.,0.));
#116429=DIRECTION('',(1.02434006807916E-22,1.4843197546388E-38,1.));
#116430=DIRECTION('center_axis',(-1.02434006807916E-22,-1.4843197546388E-38,
-1.));
#116431=DIRECTION('ref_axis',(-1.4490497842403E-16,1.,0.));
#116432=DIRECTION('',(1.02434006807916E-22,1.4843197546388E-38,1.));
#116433=DIRECTION('center_axis',(-1.02434006807916E-22,-1.4843197546388E-38,
-1.));
#116434=DIRECTION('ref_axis',(-1.4490497842403E-16,1.,0.));
#116435=DIRECTION('',(1.02434006807916E-22,1.4843197546388E-38,1.));
#116436=DIRECTION('center_axis',(-1.02434006807916E-22,-1.4843197546388E-38,
-1.));
#116437=DIRECTION('ref_axis',(-1.4490497842403E-16,1.,0.));
#116438=DIRECTION('',(1.02434006807916E-22,1.4843197546388E-38,1.));
#116439=DIRECTION('center_axis',(-4.78053475807573E-13,1.83844196516503E-12,
-1.));
#116440=DIRECTION('ref_axis',(-1.50232827312377E-11,-1.,-1.83855436624071E-12));
#116441=DIRECTION('center_axis',(0.,1.47731603554264E-17,1.));
#116442=DIRECTION('ref_axis',(0.,-1.,1.47731603554264E-17));
#116443=DIRECTION('',(0.,-1.47731603554264E-17,-1.));
#116444=DIRECTION('center_axis',(0.,1.47731603554263E-17,1.));
#116445=DIRECTION('ref_axis',(0.,-1.,1.47731603554263E-17));
#116446=DIRECTION('center_axis',(0.,1.47731603554264E-17,1.));
#116447=DIRECTION('ref_axis',(0.,-1.,1.47731603554264E-17));
#116448=DIRECTION('',(0.,-1.47731603554264E-17,-1.));
#116449=DIRECTION('center_axis',(0.,1.47731603554264E-17,1.));
#116450=DIRECTION('ref_axis',(0.,-1.,1.47731603554264E-17));
#116451=DIRECTION('',(0.,-1.47731603554264E-17,-1.));
#116452=DIRECTION('center_axis',(0.,1.47731603554264E-17,1.));
#116453=DIRECTION('ref_axis',(0.,-1.,1.47731603554264E-17));
#116454=DIRECTION('',(0.,-1.47731603554264E-17,-1.));
#116455=DIRECTION('center_axis',(0.,1.47731603554264E-17,1.));
#116456=DIRECTION('ref_axis',(0.,-1.,1.47731603554264E-17));
#116457=DIRECTION('',(0.,-1.47731603554264E-17,-1.));
#116458=DIRECTION('center_axis',(0.,1.47731603554264E-17,1.));
#116459=DIRECTION('ref_axis',(0.,-1.,1.47731603554264E-17));
#116460=DIRECTION('',(0.,-1.47731603554264E-17,-1.));
#116461=DIRECTION('center_axis',(0.,1.47731603554264E-17,1.));
#116462=DIRECTION('ref_axis',(0.,-1.,1.47731603554264E-17));
#116463=DIRECTION('',(0.,-1.47731603554264E-17,-1.));
#116464=DIRECTION('center_axis',(0.,1.47731603554264E-17,1.));
#116465=DIRECTION('ref_axis',(0.,-1.,1.47731603554264E-17));
#116466=DIRECTION('',(0.,-1.47731603554264E-17,-1.));
#116467=DIRECTION('center_axis',(0.,1.47731603554264E-17,1.));
#116468=DIRECTION('ref_axis',(0.,-1.,1.47731603554264E-17));
#116469=DIRECTION('',(0.,-1.47731603554264E-17,-1.));
#116470=DIRECTION('center_axis',(0.,1.47731603554264E-17,1.));
#116471=DIRECTION('ref_axis',(0.,-1.,1.47731603554264E-17));
#116472=DIRECTION('',(0.,-1.47731603554264E-17,-1.));
#116473=DIRECTION('center_axis',(0.,1.47731603554264E-17,1.));
#116474=DIRECTION('ref_axis',(0.,-1.,1.47731603554264E-17));
#116475=DIRECTION('',(0.,-1.47731603554264E-17,-1.));
#116476=DIRECTION('center_axis',(0.,1.47731603554264E-17,1.));
#116477=DIRECTION('ref_axis',(0.,-1.,1.47731603554264E-17));
#116478=DIRECTION('',(0.,-1.47731603554264E-17,-1.));
#116479=DIRECTION('center_axis',(0.,1.47731603554264E-17,1.));
#116480=DIRECTION('ref_axis',(0.,-1.,1.47731603554264E-17));
#116481=DIRECTION('',(0.,-1.47731603554264E-17,-1.));
#116482=DIRECTION('center_axis',(0.,1.47731603554264E-17,1.));
#116483=DIRECTION('ref_axis',(0.,-1.,1.47731603554264E-17));
#116484=DIRECTION('',(0.,-1.47731603554264E-17,-1.));
#116485=DIRECTION('center_axis',(0.,1.47731603554263E-17,1.));
#116486=DIRECTION('ref_axis',(0.,-1.,1.47731603554263E-17));
#116487=DIRECTION('center_axis',(-4.78053475807573E-13,1.83844196516503E-12,
-1.));
#116488=DIRECTION('ref_axis',(-1.50232827312377E-11,-1.,-1.83855436624071E-12));
#116489=DIRECTION('',(8.65956056235495E-17,-0.707106781186549,-0.707106781186546));
#116490=DIRECTION('center_axis',(0.,-1.47731603554264E-17,-1.));
#116491=DIRECTION('ref_axis',(0.,-1.,1.47731603554264E-17));
#116492=DIRECTION('center_axis',(0.,1.47731603554264E-17,1.));
#116493=DIRECTION('ref_axis',(0.,-1.,1.47731603554264E-17));
#116494=DIRECTION('center_axis',(0.,6.8448976313476E-17,1.));
#116495=DIRECTION('ref_axis',(0.,-1.,6.8448976313476E-17));
#116496=DIRECTION('center_axis',(0.,0.,1.));
#116497=DIRECTION('ref_axis',(-1.,0.,0.));
#116498=DIRECTION('center_axis',(0.,0.,-1.));
#116499=DIRECTION('ref_axis',(-1.,0.,0.));
#116500=DIRECTION('center_axis',(0.,6.8448976313476E-17,1.));
#116501=DIRECTION('ref_axis',(0.,-1.,6.8448976313476E-17));
#116502=DIRECTION('center_axis',(0.,6.8448976313476E-17,1.));
#116503=DIRECTION('ref_axis',(0.,-1.,6.8448976313476E-17));
#116504=DIRECTION('',(0.,-6.8448976313476E-17,-1.));
#116505=DIRECTION('center_axis',(0.,6.8448976313476E-17,1.));
#116506=DIRECTION('ref_axis',(0.,-1.,6.8448976313476E-17));
#116507=DIRECTION('center_axis',(0.,6.8448976313476E-17,1.));
#116508=DIRECTION('ref_axis',(0.,-1.,6.8448976313476E-17));
#116509=DIRECTION('',(8.65956056235493E-17,-0.707106781186548,-0.707106781186548));
#116510=DIRECTION('center_axis',(0.,6.8448976313476E-17,1.));
#116511=DIRECTION('ref_axis',(0.,-1.,6.8448976313476E-17));
#116512=DIRECTION('center_axis',(0.,6.8448976313476E-17,1.));
#116513=DIRECTION('ref_axis',(0.,-1.,6.8448976313476E-17));
#116514=DIRECTION('center_axis',(0.,-6.8448976313476E-17,-1.));
#116515=DIRECTION('ref_axis',(0.,1.,-6.8448976313476E-17));
#116516=DIRECTION('center_axis',(0.,0.,-1.));
#116517=DIRECTION('ref_axis',(-1.,0.,0.));
#116518=DIRECTION('center_axis',(0.,0.,-1.));
#116519=DIRECTION('ref_axis',(-1.,0.,0.));
#116520=DIRECTION('center_axis',(0.,0.,-1.));
#116521=DIRECTION('ref_axis',(-1.,0.,0.));
#116522=DIRECTION('center_axis',(0.,0.,-1.));
#116523=DIRECTION('ref_axis',(-1.,0.,0.));
#116524=DIRECTION('center_axis',(0.,0.,-1.));
#116525=DIRECTION('ref_axis',(-1.,0.,0.));
#116526=DIRECTION('center_axis',(0.,-6.8448976313476E-17,-1.));
#116527=DIRECTION('ref_axis',(0.,1.,-6.8448976313476E-17));
#116528=DIRECTION('center_axis',(0.,0.,1.));
#116529=DIRECTION('ref_axis',(1.,-7.6571373978539E-16,0.));
#116530=DIRECTION('center_axis',(0.,0.,1.));
#116531=DIRECTION('ref_axis',(-1.,0.,0.));
#116532=DIRECTION('center_axis',(0.,0.,1.));
#116533=DIRECTION('ref_axis',(-1.,0.,0.));
#116534=DIRECTION('center_axis',(0.,0.,1.));
#116535=DIRECTION('ref_axis',(-1.,0.,0.));
#116536=DIRECTION('center_axis',(0.,0.,1.));
#116537=DIRECTION('ref_axis',(-1.,0.,0.));
#116538=DIRECTION('center_axis',(0.,0.,1.));
#116539=DIRECTION('ref_axis',(1.,0.,0.));
#116540=DIRECTION('',(0.866025403784438,0.5,0.));
#116541=DIRECTION('',(2.50385766456193E-16,1.,0.));
#116542=DIRECTION('',(-0.866025403784439,0.5,0.));
#116543=DIRECTION('',(-0.866025403784439,-0.5,0.));
#116544=DIRECTION('',(2.50385766456193E-16,-1.,0.));
#116545=DIRECTION('',(0.866025403784438,-0.5,0.));
#116546=DIRECTION('center_axis',(1.,-2.50385766456193E-16,0.));
#116547=DIRECTION('ref_axis',(2.50385766456193E-16,1.,0.));
#116548=DIRECTION('',(0.,0.,1.));
#116549=DIRECTION('',(0.,0.,1.));
#116550=DIRECTION('center_axis',(0.5,0.866025403784439,0.));
#116551=DIRECTION('ref_axis',(-0.866025403784439,0.5,0.));
#116552=DIRECTION('',(0.,0.,1.));
#116553=DIRECTION('center_axis',(-0.5,0.866025403784439,0.));
#116554=DIRECTION('ref_axis',(-0.866025403784439,-0.5,0.));
#116555=DIRECTION('',(0.,0.,1.));
#116556=DIRECTION('center_axis',(-1.,-2.50385766456193E-16,0.));
#116557=DIRECTION('ref_axis',(2.50385766456193E-16,-1.,0.));
#116558=DIRECTION('',(0.,0.,1.));
#116559=DIRECTION('center_axis',(-0.5,-0.866025403784439,0.));
#116560=DIRECTION('ref_axis',(0.866025403784439,-0.5,0.));
#116561=DIRECTION('',(0.,0.,1.));
#116562=DIRECTION('center_axis',(0.5,-0.866025403784439,0.));
#116563=DIRECTION('ref_axis',(0.866025403784439,0.5,0.));
#116564=DIRECTION('center_axis',(0.,1.47731603554264E-17,1.));
#116565=DIRECTION('ref_axis',(0.,-1.,1.47731603554264E-17));
#116566=DIRECTION('center_axis',(-1.02434006807916E-22,-1.4843197546388E-38,
-1.));
#116567=DIRECTION('ref_axis',(-1.4490497842403E-16,1.,0.));
#368987=CARTESIAN_POINT('',(0.,0.,0.));
#368988=CARTESIAN_POINT('Origin',(1.38777878078145E-16,1.38777878078145E-16,
-4.19687500000002));
#368989=CARTESIAN_POINT('',(2.14917752421619E-17,-0.957716426222737,2.29999999999999));
#368990=CARTESIAN_POINT('',(2.14917781231183E-17,-0.957716426222737,2.35624999999998));
#368991=CARTESIAN_POINT('',(1.60269320569837E-16,-0.957716426222737,-4.19687500000002));
#368992=CARTESIAN_POINT('',(0.333926106471282,0.897615791123229,2.5));
#368993=CARTESIAN_POINT('Ctrl Pts',(-1.17286435586452E-16,-0.957716426222737,
2.29999999999999));
#368994=CARTESIAN_POINT('Ctrl Pts',(0.552937836487023,-0.957716426222737,
2.33749999999999));
#368995=CARTESIAN_POINT('Ctrl Pts',(0.829406754730535,-0.478858213111369,
2.37499999999999));
#368996=CARTESIAN_POINT('Ctrl Pts',(1.10587567297405,-3.31349931757196E-16,
2.41249999999999));
#368997=CARTESIAN_POINT('Ctrl Pts',(0.829406754730536,0.478858213111368,
2.44999999999999));
#368998=CARTESIAN_POINT('Ctrl Pts',(0.657035190041872,0.777414520932278,
2.47338032686238));
#368999=CARTESIAN_POINT('Ctrl Pts',(0.333926106471282,0.897615791123229,
2.5));
#369000=CARTESIAN_POINT('',(0.870621065093338,0.399048510926419,2.5));
#369001=CARTESIAN_POINT('Origin',(1.38778564065884E-16,1.38777878078145E-16,
2.5));
#369002=CARTESIAN_POINT('Ctrl Pts',(-1.17286435586452E-16,-0.957716426222737,
2.35624999999998));
#369003=CARTESIAN_POINT('Ctrl Pts',(0.552937836487023,-0.957716426222737,
2.39374999999998));
#369004=CARTESIAN_POINT('Ctrl Pts',(0.829406754730535,-0.478858213111369,
2.43124999999998));
#369005=CARTESIAN_POINT('Ctrl Pts',(1.07669261690991,-0.050546535823224,
2.46479163603864));
#369006=CARTESIAN_POINT('Ctrl Pts',(0.870621065093338,0.399048510926419,
2.5));
#369007=CARTESIAN_POINT('Origin',(1.38777878078145E-16,1.38777878078145E-16,
-4.19687500000002));
#369008=CARTESIAN_POINT('',(2.14917521945104E-17,-0.957716426222737,1.84999999999999));
#369009=CARTESIAN_POINT('',(2.14917550754668E-17,-0.957716426222737,1.90624999999998));
#369010=CARTESIAN_POINT('',(1.60269320569837E-16,-0.957716426222737,-4.19687500000002));
#369011=CARTESIAN_POINT('Ctrl Pts',(-1.17286435586452E-16,-0.957716426222737,
1.84999999999999));
#369012=CARTESIAN_POINT('Ctrl Pts',(0.552937836487023,-0.957716426222737,
1.88749999999999));
#369013=CARTESIAN_POINT('Ctrl Pts',(0.829406754730535,-0.478858213111369,
1.92499999999999));
#369014=CARTESIAN_POINT('Ctrl Pts',(1.10587567297405,-3.31752530400862E-16,
1.96249999999999));
#369015=CARTESIAN_POINT('Ctrl Pts',(0.829406754730536,0.478858213111368,
1.99999999999999));
#369016=CARTESIAN_POINT('Ctrl Pts',(0.552937836487024,0.957716426222737,
2.03749999999999));
#369017=CARTESIAN_POINT('Ctrl Pts',(0.,0.957716426222737,2.07499999999999));
#369018=CARTESIAN_POINT('Ctrl Pts',(-0.552937836487023,0.957716426222737,
2.11249999999999));
#369019=CARTESIAN_POINT('Ctrl Pts',(-0.829406754730535,0.478858213111368,
2.14999999999999));
#369020=CARTESIAN_POINT('Ctrl Pts',(-1.10587567297405,-6.06898104465106E-17,
2.18749999999999));
#369021=CARTESIAN_POINT('Ctrl Pts',(-0.829406754730535,-0.478858213111368,
2.22499999999999));
#369022=CARTESIAN_POINT('Ctrl Pts',(-0.552937836487024,-0.957716426222737,
2.26249999999999));
#369023=CARTESIAN_POINT('Ctrl Pts',(-1.17286435586452E-16,-0.957716426222737,
2.29999999999999));
#369024=CARTESIAN_POINT('Ctrl Pts',(-1.17286435586452E-16,-0.957716426222737,
1.90624999999998));
#369025=CARTESIAN_POINT('Ctrl Pts',(0.552937836487023,-0.957716426222737,
1.94374999999998));
#369026=CARTESIAN_POINT('Ctrl Pts',(0.829406754730535,-0.478858213111369,
1.98124999999998));
#369027=CARTESIAN_POINT('Ctrl Pts',(1.10587567297405,-3.31702205570404E-16,
2.01874999999998));
#369028=CARTESIAN_POINT('Ctrl Pts',(0.829406754730536,0.478858213111368,
2.05624999999998));
#369029=CARTESIAN_POINT('Ctrl Pts',(0.552937836487024,0.957716426222737,
2.09374999999998));
#369030=CARTESIAN_POINT('Ctrl Pts',(0.,0.957716426222737,2.13124999999998));
#369031=CARTESIAN_POINT('Ctrl Pts',(-0.552937836487023,0.957716426222737,
2.16874999999998));
#369032=CARTESIAN_POINT('Ctrl Pts',(-0.829406754730535,0.478858213111368,
2.20624999999998));
#369033=CARTESIAN_POINT('Ctrl Pts',(-1.10587567297405,-6.06394856160523E-17,
2.24374999999998));
#369034=CARTESIAN_POINT('Ctrl Pts',(-0.829406754730535,-0.478858213111368,
2.28124999999998));
#369035=CARTESIAN_POINT('Ctrl Pts',(-0.552937836487024,-0.957716426222737,
2.31874999999998));
#369036=CARTESIAN_POINT('Ctrl Pts',(-1.17286435586452E-16,-0.957716426222737,
2.35624999999998));
#369037=CARTESIAN_POINT('Origin',(1.38777878078145E-16,1.38777878078145E-16,
-4.19687500000002));
#369038=CARTESIAN_POINT('',(2.14917291468588E-17,-0.957716426222737,1.39999999999999));
#369039=CARTESIAN_POINT('',(2.14917320278152E-17,-0.957716426222737,1.45624999999998));
#369040=CARTESIAN_POINT('',(1.60269320569837E-16,-0.957716426222737,-4.19687500000002));
#369041=CARTESIAN_POINT('Ctrl Pts',(-1.17286435586452E-16,-0.957716426222737,
1.39999999999999));
#369042=CARTESIAN_POINT('Ctrl Pts',(0.552937836487023,-0.957716426222737,
1.43749999999999));
#369043=CARTESIAN_POINT('Ctrl Pts',(0.829406754730535,-0.478858213111369,
1.47499999999999));
#369044=CARTESIAN_POINT('Ctrl Pts',(1.10587567297405,-3.32155129044528E-16,
1.51249999999999));
#369045=CARTESIAN_POINT('Ctrl Pts',(0.829406754730536,0.478858213111368,
1.54999999999999));
#369046=CARTESIAN_POINT('Ctrl Pts',(0.552937836487024,0.957716426222737,
1.58749999999999));
#369047=CARTESIAN_POINT('Ctrl Pts',(0.,0.957716426222737,1.62499999999999));
#369048=CARTESIAN_POINT('Ctrl Pts',(-0.552937836487023,0.957716426222737,
1.66249999999999));
#369049=CARTESIAN_POINT('Ctrl Pts',(-0.829406754730535,0.478858213111368,
1.69999999999999));
#369050=CARTESIAN_POINT('Ctrl Pts',(-1.10587567297405,-6.10924090901767E-17,
1.73749999999999));
#369051=CARTESIAN_POINT('Ctrl Pts',(-0.829406754730535,-0.478858213111368,
1.77499999999999));
#369052=CARTESIAN_POINT('Ctrl Pts',(-0.552937836487024,-0.957716426222737,
1.81249999999999));
#369053=CARTESIAN_POINT('Ctrl Pts',(-1.17286435586452E-16,-0.957716426222737,
1.84999999999999));
#369054=CARTESIAN_POINT('Ctrl Pts',(-1.17286435586452E-16,-0.957716426222737,
1.45624999999998));
#369055=CARTESIAN_POINT('Ctrl Pts',(0.552937836487023,-0.957716426222737,
1.49374999999998));
#369056=CARTESIAN_POINT('Ctrl Pts',(0.829406754730535,-0.478858213111369,
1.53124999999998));
#369057=CARTESIAN_POINT('Ctrl Pts',(1.10587567297405,-3.3210480421407E-16,
1.56874999999998));
#369058=CARTESIAN_POINT('Ctrl Pts',(0.829406754730536,0.478858213111368,
1.60624999999998));
#369059=CARTESIAN_POINT('Ctrl Pts',(0.552937836487024,0.957716426222737,
1.64374999999998));
#369060=CARTESIAN_POINT('Ctrl Pts',(0.,0.957716426222737,1.68124999999998));
#369061=CARTESIAN_POINT('Ctrl Pts',(-0.552937836487023,0.957716426222737,
1.71874999999998));
#369062=CARTESIAN_POINT('Ctrl Pts',(-0.829406754730535,0.478858213111368,
1.75624999999998));
#369063=CARTESIAN_POINT('Ctrl Pts',(-1.10587567297405,-6.10420842597184E-17,
1.79374999999998));
#369064=CARTESIAN_POINT('Ctrl Pts',(-0.829406754730535,-0.478858213111368,
1.83124999999998));
#369065=CARTESIAN_POINT('Ctrl Pts',(-0.552937836487024,-0.957716426222737,
1.86874999999998));
#369066=CARTESIAN_POINT('Ctrl Pts',(-1.17286435586452E-16,-0.957716426222737,
1.90624999999998));
#369067=CARTESIAN_POINT('Origin',(1.38777878078145E-16,1.38777878078145E-16,
-4.19687500000002));
#369068=CARTESIAN_POINT('',(2.14917060992073E-17,-0.957716426222737,0.949999999999986));
#369069=CARTESIAN_POINT('',(2.14917089801637E-17,-0.957716426222737,1.00624999999998));
#369070=CARTESIAN_POINT('',(1.60269320569837E-16,-0.957716426222737,-4.19687500000002));
#369071=CARTESIAN_POINT('Ctrl Pts',(-1.17286435586452E-16,-0.957716426222737,
0.949999999999986));
#369072=CARTESIAN_POINT('Ctrl Pts',(0.552937836487023,-0.957716426222737,
0.987499999999986));
#369073=CARTESIAN_POINT('Ctrl Pts',(0.829406754730535,-0.478858213111369,
1.02499999999999));
#369074=CARTESIAN_POINT('Ctrl Pts',(1.10587567297405,-3.32557727688194E-16,
1.06249999999999));
#369075=CARTESIAN_POINT('Ctrl Pts',(0.829406754730536,0.478858213111368,
1.09999999999999));
#369076=CARTESIAN_POINT('Ctrl Pts',(0.552937836487024,0.957716426222737,
1.13749999999999));
#369077=CARTESIAN_POINT('Ctrl Pts',(0.,0.957716426222737,1.17499999999999));
#369078=CARTESIAN_POINT('Ctrl Pts',(-0.552937836487023,0.957716426222737,
1.21249999999999));
#369079=CARTESIAN_POINT('Ctrl Pts',(-0.829406754730535,0.478858213111368,
1.24999999999999));
#369080=CARTESIAN_POINT('Ctrl Pts',(-1.10587567297405,-6.14950077338427E-17,
1.28749999999999));
#369081=CARTESIAN_POINT('Ctrl Pts',(-0.829406754730535,-0.478858213111368,
1.32499999999999));
#369082=CARTESIAN_POINT('Ctrl Pts',(-0.552937836487024,-0.957716426222737,
1.36249999999999));
#369083=CARTESIAN_POINT('Ctrl Pts',(-1.17286435586452E-16,-0.957716426222737,
1.39999999999999));
#369084=CARTESIAN_POINT('Ctrl Pts',(-1.17286435586452E-16,-0.957716426222737,
1.00624999999998));
#369085=CARTESIAN_POINT('Ctrl Pts',(0.552937836487023,-0.957716426222737,
1.04374999999998));
#369086=CARTESIAN_POINT('Ctrl Pts',(0.829406754730535,-0.478858213111369,
1.08124999999998));
#369087=CARTESIAN_POINT('Ctrl Pts',(1.10587567297405,-3.32507402857736E-16,
1.11874999999998));
#369088=CARTESIAN_POINT('Ctrl Pts',(0.829406754730536,0.478858213111368,
1.15624999999998));
#369089=CARTESIAN_POINT('Ctrl Pts',(0.552937836487024,0.957716426222737,
1.19374999999998));
#369090=CARTESIAN_POINT('Ctrl Pts',(0.,0.957716426222737,1.23124999999998));
#369091=CARTESIAN_POINT('Ctrl Pts',(-0.552937836487023,0.957716426222737,
1.26874999999998));
#369092=CARTESIAN_POINT('Ctrl Pts',(-0.829406754730535,0.478858213111368,
1.30624999999998));
#369093=CARTESIAN_POINT('Ctrl Pts',(-1.10587567297405,-6.14446829033844E-17,
1.34374999999998));
#369094=CARTESIAN_POINT('Ctrl Pts',(-0.829406754730535,-0.478858213111368,
1.38124999999998));
#369095=CARTESIAN_POINT('Ctrl Pts',(-0.552937836487024,-0.957716426222737,
1.41874999999998));
#369096=CARTESIAN_POINT('Ctrl Pts',(-1.17286435586452E-16,-0.957716426222737,
1.45624999999998));
#369097=CARTESIAN_POINT('Origin',(1.38777878078145E-16,1.38777878078145E-16,
-4.19687500000002));
#369098=CARTESIAN_POINT('',(2.14916830515557E-17,-0.957716426222737,0.499999999999986));
#369099=CARTESIAN_POINT('',(2.14916859325122E-17,-0.957716426222737,0.556249999999979));
#369100=CARTESIAN_POINT('',(1.60269320569837E-16,-0.957716426222737,-4.19687500000002));
#369101=CARTESIAN_POINT('Ctrl Pts',(-1.17286435586452E-16,-0.957716426222737,
0.499999999999986));
#369102=CARTESIAN_POINT('Ctrl Pts',(0.552937836487023,-0.957716426222737,
0.537499999999986));
#369103=CARTESIAN_POINT('Ctrl Pts',(0.829406754730535,-0.478858213111369,
0.574999999999986));
#369104=CARTESIAN_POINT('Ctrl Pts',(1.10587567297405,-3.3296032633186E-16,
0.612499999999986));
#369105=CARTESIAN_POINT('Ctrl Pts',(0.829406754730536,0.478858213111368,
0.649999999999987));
#369106=CARTESIAN_POINT('Ctrl Pts',(0.552937836487024,0.957716426222737,
0.687499999999986));
#369107=CARTESIAN_POINT('Ctrl Pts',(0.,0.957716426222737,0.724999999999986));
#369108=CARTESIAN_POINT('Ctrl Pts',(-0.552937836487023,0.957716426222737,
0.762499999999986));
#369109=CARTESIAN_POINT('Ctrl Pts',(-0.829406754730535,0.478858213111368,
0.799999999999986));
#369110=CARTESIAN_POINT('Ctrl Pts',(-1.10587567297405,-6.18976063775088E-17,
0.837499999999986));
#369111=CARTESIAN_POINT('Ctrl Pts',(-0.829406754730535,-0.478858213111368,
0.874999999999986));
#369112=CARTESIAN_POINT('Ctrl Pts',(-0.552937836487024,-0.957716426222737,
0.912499999999986));
#369113=CARTESIAN_POINT('Ctrl Pts',(-1.17286435586452E-16,-0.957716426222737,
0.949999999999986));
#369114=CARTESIAN_POINT('Ctrl Pts',(-1.17286435586452E-16,-0.957716426222737,
0.556249999999979));
#369115=CARTESIAN_POINT('Ctrl Pts',(0.552937836487023,-0.957716426222737,
0.59374999999998));
#369116=CARTESIAN_POINT('Ctrl Pts',(0.829406754730535,-0.478858213111369,
0.63124999999998));
#369117=CARTESIAN_POINT('Ctrl Pts',(1.10587567297405,-3.32910001501402E-16,
0.66874999999998));
#369118=CARTESIAN_POINT('Ctrl Pts',(0.829406754730536,0.478858213111368,
0.70624999999998));
#369119=CARTESIAN_POINT('Ctrl Pts',(0.552937836487024,0.957716426222737,
0.74374999999998));
#369120=CARTESIAN_POINT('Ctrl Pts',(0.,0.957716426222737,0.78124999999998));
#369121=CARTESIAN_POINT('Ctrl Pts',(-0.552937836487023,0.957716426222737,
0.81874999999998));
#369122=CARTESIAN_POINT('Ctrl Pts',(-0.829406754730535,0.478858213111368,
0.85624999999998));
#369123=CARTESIAN_POINT('Ctrl Pts',(-1.10587567297405,-6.18472815470505E-17,
0.89374999999998));
#369124=CARTESIAN_POINT('Ctrl Pts',(-0.829406754730535,-0.478858213111368,
0.93124999999998));
#369125=CARTESIAN_POINT('Ctrl Pts',(-0.552937836487024,-0.957716426222737,
0.96874999999998));
#369126=CARTESIAN_POINT('Ctrl Pts',(-1.17286435586452E-16,-0.957716426222737,
1.00624999999998));
#369127=CARTESIAN_POINT('Origin',(1.38777878078145E-16,1.38777878078145E-16,
-4.19687500000002));
#369128=CARTESIAN_POINT('',(2.14916600039042E-17,-0.957716426222737,0.0499999999999858));
#369129=CARTESIAN_POINT('',(2.14916628848607E-17,-0.957716426222737,0.10624999999998));
#369130=CARTESIAN_POINT('',(1.60269320569837E-16,-0.957716426222737,-4.19687500000002));
#369131=CARTESIAN_POINT('Ctrl Pts',(-1.17286435586452E-16,-0.957716426222737,
0.0499999999999858));
#369132=CARTESIAN_POINT('Ctrl Pts',(0.552937836487023,-0.957716426222737,
0.087499999999986));
#369133=CARTESIAN_POINT('Ctrl Pts',(0.829406754730535,-0.478858213111369,
0.124999999999986));
#369134=CARTESIAN_POINT('Ctrl Pts',(1.10587567297405,-3.33362924975526E-16,
0.162499999999987));
#369135=CARTESIAN_POINT('Ctrl Pts',(0.829406754730536,0.478858213111368,
0.199999999999986));
#369136=CARTESIAN_POINT('Ctrl Pts',(0.552937836487024,0.957716426222737,
0.237499999999986));
#369137=CARTESIAN_POINT('Ctrl Pts',(0.,0.957716426222737,0.274999999999986));
#369138=CARTESIAN_POINT('Ctrl Pts',(-0.552937836487023,0.957716426222737,
0.312499999999986));
#369139=CARTESIAN_POINT('Ctrl Pts',(-0.829406754730535,0.478858213111368,
0.349999999999986));
#369140=CARTESIAN_POINT('Ctrl Pts',(-1.10587567297405,-6.23002050211748E-17,
0.387499999999986));
#369141=CARTESIAN_POINT('Ctrl Pts',(-0.829406754730535,-0.478858213111368,
0.424999999999986));
#369142=CARTESIAN_POINT('Ctrl Pts',(-0.552937836487024,-0.957716426222737,
0.462499999999986));
#369143=CARTESIAN_POINT('Ctrl Pts',(-1.17286435586452E-16,-0.957716426222737,
0.499999999999986));
#369144=CARTESIAN_POINT('Ctrl Pts',(-1.17286435586452E-16,-0.957716426222737,
0.10624999999998));
#369145=CARTESIAN_POINT('Ctrl Pts',(0.552937836487023,-0.957716426222737,
0.14374999999998));
#369146=CARTESIAN_POINT('Ctrl Pts',(0.829406754730535,-0.478858213111369,
0.18124999999998));
#369147=CARTESIAN_POINT('Ctrl Pts',(1.10587567297405,-3.33312600145068E-16,
0.21874999999998));
#369148=CARTESIAN_POINT('Ctrl Pts',(0.829406754730536,0.478858213111368,
0.25624999999998));
#369149=CARTESIAN_POINT('Ctrl Pts',(0.552937836487024,0.957716426222737,
0.29374999999998));
#369150=CARTESIAN_POINT('Ctrl Pts',(0.,0.957716426222737,0.33124999999998));
#369151=CARTESIAN_POINT('Ctrl Pts',(-0.552937836487023,0.957716426222737,
0.36874999999998));
#369152=CARTESIAN_POINT('Ctrl Pts',(-0.829406754730535,0.478858213111368,
0.40624999999998));
#369153=CARTESIAN_POINT('Ctrl Pts',(-1.10587567297405,-6.22498801907165E-17,
0.44374999999998));
#369154=CARTESIAN_POINT('Ctrl Pts',(-0.829406754730535,-0.478858213111368,
0.48124999999998));
#369155=CARTESIAN_POINT('Ctrl Pts',(-0.552937836487024,-0.957716426222737,
0.51874999999998));
#369156=CARTESIAN_POINT('Ctrl Pts',(-1.17286435586452E-16,-0.957716426222737,
0.556249999999979));
#369157=CARTESIAN_POINT('Origin',(1.38777878078145E-16,1.38777878078145E-16,
-4.19687500000002));
#369158=CARTESIAN_POINT('',(2.14916369562527E-17,-0.957716426222737,-0.400000000000014));
#369159=CARTESIAN_POINT('',(2.14916398372091E-17,-0.957716426222737,-0.34375000000002));
#369160=CARTESIAN_POINT('',(1.60269320569837E-16,-0.957716426222737,-4.19687500000002));
#369161=CARTESIAN_POINT('Ctrl Pts',(-1.17286435586452E-16,-0.957716426222737,
-0.400000000000014));
#369162=CARTESIAN_POINT('Ctrl Pts',(0.552937836487023,-0.957716426222737,
-0.362500000000014));
#369163=CARTESIAN_POINT('Ctrl Pts',(0.829406754730535,-0.478858213111369,
-0.325000000000014));
#369164=CARTESIAN_POINT('Ctrl Pts',(1.10587567297405,-3.33765523619192E-16,
-0.287500000000013));
#369165=CARTESIAN_POINT('Ctrl Pts',(0.829406754730536,0.478858213111368,
-0.250000000000014));
#369166=CARTESIAN_POINT('Ctrl Pts',(0.552937836487024,0.957716426222737,
-0.212500000000014));
#369167=CARTESIAN_POINT('Ctrl Pts',(0.,0.957716426222737,-0.175000000000014));
#369168=CARTESIAN_POINT('Ctrl Pts',(-0.552937836487023,0.957716426222737,
-0.137500000000013));
#369169=CARTESIAN_POINT('Ctrl Pts',(-0.829406754730535,0.478858213111368,
-0.100000000000014));
#369170=CARTESIAN_POINT('Ctrl Pts',(-1.10587567297405,-6.27028036648408E-17,
-0.0625000000000139));
#369171=CARTESIAN_POINT('Ctrl Pts',(-0.829406754730535,-0.478858213111368,
-0.0250000000000137));
#369172=CARTESIAN_POINT('Ctrl Pts',(-0.552937836487024,-0.957716426222737,
0.0124999999999865));
#369173=CARTESIAN_POINT('Ctrl Pts',(-1.17286435586452E-16,-0.957716426222737,
0.0499999999999858));
#369174=CARTESIAN_POINT('Ctrl Pts',(-1.17286435586452E-16,-0.957716426222737,
-0.34375000000002));
#369175=CARTESIAN_POINT('Ctrl Pts',(0.552937836487023,-0.957716426222737,
-0.30625000000002));
#369176=CARTESIAN_POINT('Ctrl Pts',(0.829406754730535,-0.478858213111369,
-0.26875000000002));
#369177=CARTESIAN_POINT('Ctrl Pts',(1.10587567297405,-3.33715198788734E-16,
-0.23125000000002));
#369178=CARTESIAN_POINT('Ctrl Pts',(0.829406754730536,0.478858213111368,
-0.19375000000002));
#369179=CARTESIAN_POINT('Ctrl Pts',(0.552937836487024,0.957716426222737,
-0.15625000000002));
#369180=CARTESIAN_POINT('Ctrl Pts',(0.,0.957716426222737,-0.11875000000002));
#369181=CARTESIAN_POINT('Ctrl Pts',(-0.552937836487023,0.957716426222737,
-0.0812500000000197));
#369182=CARTESIAN_POINT('Ctrl Pts',(-0.829406754730535,0.478858213111368,
-0.0437500000000203));
#369183=CARTESIAN_POINT('Ctrl Pts',(-1.10587567297405,-6.26524788343826E-17,
-0.00625000000002013));
#369184=CARTESIAN_POINT('Ctrl Pts',(-0.829406754730535,-0.478858213111368,
0.0312499999999801));
#369185=CARTESIAN_POINT('Ctrl Pts',(-0.552937836487024,-0.957716426222737,
0.0687499999999803));
#369186=CARTESIAN_POINT('Ctrl Pts',(-1.17286435586452E-16,-0.957716426222737,
0.10624999999998));
#369187=CARTESIAN_POINT('Origin',(1.38777878078145E-16,1.38777878078145E-16,
-4.19687500000002));
#369188=CARTESIAN_POINT('',(2.14916139086011E-17,-0.957716426222737,-0.850000000000014));
#369189=CARTESIAN_POINT('',(2.14916167895576E-17,-0.957716426222737,-0.79375000000002));
#369190=CARTESIAN_POINT('',(1.60269320569837E-16,-0.957716426222737,-4.19687500000002));
#369191=CARTESIAN_POINT('Ctrl Pts',(-1.17286435586452E-16,-0.957716426222737,
-0.850000000000014));
#369192=CARTESIAN_POINT('Ctrl Pts',(0.552937836487023,-0.957716426222737,
-0.812500000000014));
#369193=CARTESIAN_POINT('Ctrl Pts',(0.829406754730535,-0.478858213111369,
-0.775000000000014));
#369194=CARTESIAN_POINT('Ctrl Pts',(1.10587567297405,-3.34168122262858E-16,
-0.737500000000014));
#369195=CARTESIAN_POINT('Ctrl Pts',(0.829406754730536,0.478858213111368,
-0.700000000000014));
#369196=CARTESIAN_POINT('Ctrl Pts',(0.552937836487024,0.957716426222737,
-0.662500000000014));
#369197=CARTESIAN_POINT('Ctrl Pts',(0.,0.957716426222737,-0.625000000000014));
#369198=CARTESIAN_POINT('Ctrl Pts',(-0.552937836487023,0.957716426222737,
-0.587500000000014));
#369199=CARTESIAN_POINT('Ctrl Pts',(-0.829406754730535,0.478858213111368,
-0.550000000000014));
#369200=CARTESIAN_POINT('Ctrl Pts',(-1.10587567297405,-6.31054023085069E-17,
-0.512500000000014));
#369201=CARTESIAN_POINT('Ctrl Pts',(-0.829406754730535,-0.478858213111368,
-0.475000000000014));
#369202=CARTESIAN_POINT('Ctrl Pts',(-0.552937836487024,-0.957716426222737,
-0.437500000000014));
#369203=CARTESIAN_POINT('Ctrl Pts',(-1.17286435586452E-16,-0.957716426222737,
-0.400000000000014));
#369204=CARTESIAN_POINT('Ctrl Pts',(-1.17286435586452E-16,-0.957716426222737,
-0.79375000000002));
#369205=CARTESIAN_POINT('Ctrl Pts',(0.552937836487023,-0.957716426222737,
-0.75625000000002));
#369206=CARTESIAN_POINT('Ctrl Pts',(0.829406754730535,-0.478858213111369,
-0.71875000000002));
#369207=CARTESIAN_POINT('Ctrl Pts',(1.10587567297405,-3.341177974324E-16,
-0.68125000000002));
#369208=CARTESIAN_POINT('Ctrl Pts',(0.829406754730536,0.478858213111368,
-0.64375000000002));
#369209=CARTESIAN_POINT('Ctrl Pts',(0.552937836487024,0.957716426222737,
-0.60625000000002));
#369210=CARTESIAN_POINT('Ctrl Pts',(0.,0.957716426222737,-0.56875000000002));
#369211=CARTESIAN_POINT('Ctrl Pts',(-0.552937836487023,0.957716426222737,
-0.53125000000002));
#369212=CARTESIAN_POINT('Ctrl Pts',(-0.829406754730535,0.478858213111368,
-0.49375000000002));
#369213=CARTESIAN_POINT('Ctrl Pts',(-1.10587567297405,-6.30550774780486E-17,
-0.45625000000002));
#369214=CARTESIAN_POINT('Ctrl Pts',(-0.829406754730535,-0.478858213111368,
-0.41875000000002));
#369215=CARTESIAN_POINT('Ctrl Pts',(-0.552937836487024,-0.957716426222737,
-0.38125000000002));
#369216=CARTESIAN_POINT('Ctrl Pts',(-1.17286435586452E-16,-0.957716426222737,
-0.34375000000002));
#369217=CARTESIAN_POINT('Origin',(1.38777878078145E-16,1.38777878078145E-16,
-4.19687500000002));
#369218=CARTESIAN_POINT('',(2.14915908609496E-17,-0.957716426222737,-1.30000000000001));
#369219=CARTESIAN_POINT('',(2.14915937419061E-17,-0.957716426222737,-1.24375000000002));
#369220=CARTESIAN_POINT('',(1.60269320569837E-16,-0.957716426222737,-4.19687500000002));
#369221=CARTESIAN_POINT('Ctrl Pts',(-1.17286435586452E-16,-0.957716426222737,
-1.30000000000001));
#369222=CARTESIAN_POINT('Ctrl Pts',(0.552937836487023,-0.957716426222737,
-1.26250000000001));
#369223=CARTESIAN_POINT('Ctrl Pts',(0.829406754730535,-0.478858213111369,
-1.22500000000001));
#369224=CARTESIAN_POINT('Ctrl Pts',(1.10587567297405,-3.34570720906524E-16,
-1.18750000000001));
#369225=CARTESIAN_POINT('Ctrl Pts',(0.829406754730536,0.478858213111368,
-1.15000000000001));
#369226=CARTESIAN_POINT('Ctrl Pts',(0.552937836487024,0.957716426222737,
-1.11250000000001));
#369227=CARTESIAN_POINT('Ctrl Pts',(0.,0.957716426222737,-1.07500000000001));
#369228=CARTESIAN_POINT('Ctrl Pts',(-0.552937836487023,0.957716426222737,
-1.03750000000001));
#369229=CARTESIAN_POINT('Ctrl Pts',(-0.829406754730535,0.478858213111368,
-1.00000000000001));
#369230=CARTESIAN_POINT('Ctrl Pts',(-1.10587567297405,-6.35080009521729E-17,
-0.962500000000014));
#369231=CARTESIAN_POINT('Ctrl Pts',(-0.829406754730535,-0.478858213111368,
-0.925000000000014));
#369232=CARTESIAN_POINT('Ctrl Pts',(-0.552937836487024,-0.957716426222737,
-0.887500000000014));
#369233=CARTESIAN_POINT('Ctrl Pts',(-1.17286435586452E-16,-0.957716426222737,
-0.850000000000014));
#369234=CARTESIAN_POINT('Ctrl Pts',(-1.17286435586452E-16,-0.957716426222737,
-1.24375000000002));
#369235=CARTESIAN_POINT('Ctrl Pts',(0.552937836487023,-0.957716426222737,
-1.20625000000002));
#369236=CARTESIAN_POINT('Ctrl Pts',(0.829406754730535,-0.478858213111369,
-1.16875000000002));
#369237=CARTESIAN_POINT('Ctrl Pts',(1.10587567297405,-3.34520396076066E-16,
-1.13125000000002));
#369238=CARTESIAN_POINT('Ctrl Pts',(0.829406754730536,0.478858213111368,
-1.09375000000002));
#369239=CARTESIAN_POINT('Ctrl Pts',(0.552937836487024,0.957716426222737,
-1.05625000000002));
#369240=CARTESIAN_POINT('Ctrl Pts',(0.,0.957716426222737,-1.01875000000002));
#369241=CARTESIAN_POINT('Ctrl Pts',(-0.552937836487023,0.957716426222737,
-0.98125000000002));
#369242=CARTESIAN_POINT('Ctrl Pts',(-0.829406754730535,0.478858213111368,
-0.94375000000002));
#369243=CARTESIAN_POINT('Ctrl Pts',(-1.10587567297405,-6.34576761217147E-17,
-0.90625000000002));
#369244=CARTESIAN_POINT('Ctrl Pts',(-0.829406754730535,-0.478858213111368,
-0.86875000000002));
#369245=CARTESIAN_POINT('Ctrl Pts',(-0.552937836487024,-0.957716426222737,
-0.83125000000002));
#369246=CARTESIAN_POINT('Ctrl Pts',(-1.17286435586452E-16,-0.957716426222737,
-0.79375000000002));
#369247=CARTESIAN_POINT('Origin',(1.38777878078145E-16,1.38777878078145E-16,
-4.19687500000002));
#369248=CARTESIAN_POINT('',(2.14915678132981E-17,-0.957716426222737,-1.75000000000001));
#369249=CARTESIAN_POINT('',(2.14915706942545E-17,-0.957716426222737,-1.69375000000002));
#369250=CARTESIAN_POINT('',(1.60269320569837E-16,-0.957716426222737,-4.19687500000002));
#369251=CARTESIAN_POINT('Ctrl Pts',(-1.17286435586452E-16,-0.957716426222737,
-1.75000000000001));
#369252=CARTESIAN_POINT('Ctrl Pts',(0.552937836487023,-0.957716426222737,
-1.71250000000001));
#369253=CARTESIAN_POINT('Ctrl Pts',(0.829406754730535,-0.478858213111369,
-1.67500000000001));
#369254=CARTESIAN_POINT('Ctrl Pts',(1.10587567297405,-3.3497331955019E-16,
-1.63750000000001));
#369255=CARTESIAN_POINT('Ctrl Pts',(0.829406754730536,0.478858213111368,
-1.60000000000001));
#369256=CARTESIAN_POINT('Ctrl Pts',(0.552937836487024,0.957716426222737,
-1.56250000000001));
#369257=CARTESIAN_POINT('Ctrl Pts',(0.,0.957716426222737,-1.52500000000001));
#369258=CARTESIAN_POINT('Ctrl Pts',(-0.552937836487023,0.957716426222737,
-1.48750000000001));
#369259=CARTESIAN_POINT('Ctrl Pts',(-0.829406754730535,0.478858213111368,
-1.45000000000001));
#369260=CARTESIAN_POINT('Ctrl Pts',(-1.10587567297405,-6.3910599595839E-17,
-1.41250000000001));
#369261=CARTESIAN_POINT('Ctrl Pts',(-0.829406754730535,-0.478858213111368,
-1.37500000000001));
#369262=CARTESIAN_POINT('Ctrl Pts',(-0.552937836487024,-0.957716426222737,
-1.33750000000001));
#369263=CARTESIAN_POINT('Ctrl Pts',(-1.17286435586452E-16,-0.957716426222737,
-1.30000000000001));
#369264=CARTESIAN_POINT('Ctrl Pts',(-1.17286435586452E-16,-0.957716426222737,
-1.69375000000002));
#369265=CARTESIAN_POINT('Ctrl Pts',(0.552937836487023,-0.957716426222737,
-1.65625000000002));
#369266=CARTESIAN_POINT('Ctrl Pts',(0.829406754730535,-0.478858213111369,
-1.61875000000002));
#369267=CARTESIAN_POINT('Ctrl Pts',(1.10587567297405,-3.34922994719732E-16,
-1.58125000000002));
#369268=CARTESIAN_POINT('Ctrl Pts',(0.829406754730536,0.478858213111368,
-1.54375000000002));
#369269=CARTESIAN_POINT('Ctrl Pts',(0.552937836487024,0.957716426222737,
-1.50625000000002));
#369270=CARTESIAN_POINT('Ctrl Pts',(0.,0.957716426222737,-1.46875000000002));
#369271=CARTESIAN_POINT('Ctrl Pts',(-0.552937836487023,0.957716426222737,
-1.43125000000002));
#369272=CARTESIAN_POINT('Ctrl Pts',(-0.829406754730535,0.478858213111368,
-1.39375000000002));
#369273=CARTESIAN_POINT('Ctrl Pts',(-1.10587567297405,-6.38602747653807E-17,
-1.35625000000002));
#369274=CARTESIAN_POINT('Ctrl Pts',(-0.829406754730535,-0.478858213111368,
-1.31875000000002));
#369275=CARTESIAN_POINT('Ctrl Pts',(-0.552937836487024,-0.957716426222737,
-1.28125000000002));
#369276=CARTESIAN_POINT('Ctrl Pts',(-1.17286435586452E-16,-0.957716426222737,
-1.24375000000002));
#369277=CARTESIAN_POINT('Origin',(1.38777878078145E-16,1.38777878078145E-16,
-4.19687500000002));
#369278=CARTESIAN_POINT('',(2.14915447656466E-17,-0.957716426222737,-2.20000000000001));
#369279=CARTESIAN_POINT('',(2.1491547646603E-17,-0.957716426222737,-2.14375000000002));
#369280=CARTESIAN_POINT('',(1.60269320569837E-16,-0.957716426222737,-4.19687500000002));
#369281=CARTESIAN_POINT('Ctrl Pts',(-1.17286435586452E-16,-0.957716426222737,
-2.20000000000001));
#369282=CARTESIAN_POINT('Ctrl Pts',(0.552937836487023,-0.957716426222737,
-2.16250000000001));
#369283=CARTESIAN_POINT('Ctrl Pts',(0.829406754730535,-0.478858213111369,
-2.12500000000001));
#369284=CARTESIAN_POINT('Ctrl Pts',(1.10587567297405,-3.35375918193856E-16,
-2.08750000000001));
#369285=CARTESIAN_POINT('Ctrl Pts',(0.829406754730536,0.478858213111368,
-2.05000000000001));
#369286=CARTESIAN_POINT('Ctrl Pts',(0.552937836487024,0.957716426222737,
-2.01250000000001));
#369287=CARTESIAN_POINT('Ctrl Pts',(0.,0.957716426222737,-1.97500000000001));
#369288=CARTESIAN_POINT('Ctrl Pts',(-0.552937836487023,0.957716426222737,
-1.93750000000001));
#369289=CARTESIAN_POINT('Ctrl Pts',(-0.829406754730535,0.478858213111368,
-1.90000000000001));
#369290=CARTESIAN_POINT('Ctrl Pts',(-1.10587567297405,-6.4313198239505E-17,
-1.86250000000001));
#369291=CARTESIAN_POINT('Ctrl Pts',(-0.829406754730535,-0.478858213111368,
-1.82500000000001));
#369292=CARTESIAN_POINT('Ctrl Pts',(-0.552937836487024,-0.957716426222737,
-1.78750000000001));
#369293=CARTESIAN_POINT('Ctrl Pts',(-1.17286435586452E-16,-0.957716426222737,
-1.75000000000001));
#369294=CARTESIAN_POINT('Ctrl Pts',(-1.17286435586452E-16,-0.957716426222737,
-2.14375000000002));
#369295=CARTESIAN_POINT('Ctrl Pts',(0.552937836487023,-0.957716426222737,
-2.10625000000002));
#369296=CARTESIAN_POINT('Ctrl Pts',(0.829406754730535,-0.478858213111369,
-2.06875000000002));
#369297=CARTESIAN_POINT('Ctrl Pts',(1.10587567297405,-3.35325593363398E-16,
-2.03125000000002));
#369298=CARTESIAN_POINT('Ctrl Pts',(0.829406754730536,0.478858213111368,
-1.99375000000002));
#369299=CARTESIAN_POINT('Ctrl Pts',(0.552937836487024,0.957716426222737,
-1.95625000000002));
#369300=CARTESIAN_POINT('Ctrl Pts',(0.,0.957716426222737,-1.91875000000002));
#369301=CARTESIAN_POINT('Ctrl Pts',(-0.552937836487023,0.957716426222737,
-1.88125000000002));
#369302=CARTESIAN_POINT('Ctrl Pts',(-0.829406754730535,0.478858213111368,
-1.84375000000002));
#369303=CARTESIAN_POINT('Ctrl Pts',(-1.10587567297405,-6.42628734090468E-17,
-1.80625000000002));
#369304=CARTESIAN_POINT('Ctrl Pts',(-0.829406754730535,-0.478858213111368,
-1.76875000000002));
#369305=CARTESIAN_POINT('Ctrl Pts',(-0.552937836487024,-0.957716426222737,
-1.73125000000002));
#369306=CARTESIAN_POINT('Ctrl Pts',(-1.17286435586452E-16,-0.957716426222737,
-1.69375000000002));
#369307=CARTESIAN_POINT('Origin',(1.38777878078145E-16,1.38777878078145E-16,
-4.19687500000002));
#369308=CARTESIAN_POINT('',(2.1491521717995E-17,-0.957716426222737,-2.65000000000001));
#369309=CARTESIAN_POINT('',(2.14915245989515E-17,-0.957716426222737,-2.59375000000002));
#369310=CARTESIAN_POINT('',(1.60269320569837E-16,-0.957716426222737,-4.19687500000002));
#369311=CARTESIAN_POINT('Ctrl Pts',(-1.17286435586452E-16,-0.957716426222737,
-2.65000000000001));
#369312=CARTESIAN_POINT('Ctrl Pts',(0.552937836487023,-0.957716426222737,
-2.61250000000001));
#369313=CARTESIAN_POINT('Ctrl Pts',(0.829406754730535,-0.478858213111369,
-2.57500000000001));
#369314=CARTESIAN_POINT('Ctrl Pts',(1.10587567297405,-3.35778516837522E-16,
-2.53750000000001));
#369315=CARTESIAN_POINT('Ctrl Pts',(0.829406754730536,0.478858213111368,
-2.50000000000001));
#369316=CARTESIAN_POINT('Ctrl Pts',(0.552937836487024,0.957716426222737,
-2.46250000000001));
#369317=CARTESIAN_POINT('Ctrl Pts',(0.,0.957716426222737,-2.42500000000001));
#369318=CARTESIAN_POINT('Ctrl Pts',(-0.552937836487023,0.957716426222737,
-2.38750000000001));
#369319=CARTESIAN_POINT('Ctrl Pts',(-0.829406754730535,0.478858213111368,
-2.35000000000001));
#369320=CARTESIAN_POINT('Ctrl Pts',(-1.10587567297405,-6.47157968831711E-17,
-2.31250000000001));
#369321=CARTESIAN_POINT('Ctrl Pts',(-0.829406754730535,-0.478858213111368,
-2.27500000000001));
#369322=CARTESIAN_POINT('Ctrl Pts',(-0.552937836487024,-0.957716426222737,
-2.23750000000001));
#369323=CARTESIAN_POINT('Ctrl Pts',(-1.17286435586452E-16,-0.957716426222737,
-2.20000000000001));
#369324=CARTESIAN_POINT('Ctrl Pts',(-1.17286435586452E-16,-0.957716426222737,
-2.59375000000002));
#369325=CARTESIAN_POINT('Ctrl Pts',(0.552937836487023,-0.957716426222737,
-2.55625000000002));
#369326=CARTESIAN_POINT('Ctrl Pts',(0.829406754730535,-0.478858213111369,
-2.51875000000002));
#369327=CARTESIAN_POINT('Ctrl Pts',(1.10587567297405,-3.35728192007064E-16,
-2.48125000000002));
#369328=CARTESIAN_POINT('Ctrl Pts',(0.829406754730536,0.478858213111368,
-2.44375000000002));
#369329=CARTESIAN_POINT('Ctrl Pts',(0.552937836487024,0.957716426222737,
-2.40625000000002));
#369330=CARTESIAN_POINT('Ctrl Pts',(0.,0.957716426222737,-2.36875000000002));
#369331=CARTESIAN_POINT('Ctrl Pts',(-0.552937836487023,0.957716426222737,
-2.33125000000002));
#369332=CARTESIAN_POINT('Ctrl Pts',(-0.829406754730535,0.478858213111368,
-2.29375000000002));
#369333=CARTESIAN_POINT('Ctrl Pts',(-1.10587567297405,-6.46654720527128E-17,
-2.25625000000002));
#369334=CARTESIAN_POINT('Ctrl Pts',(-0.829406754730535,-0.478858213111368,
-2.21875000000002));
#369335=CARTESIAN_POINT('Ctrl Pts',(-0.552937836487024,-0.957716426222737,
-2.18125000000002));
#369336=CARTESIAN_POINT('Ctrl Pts',(-1.17286435586452E-16,-0.957716426222737,
-2.14375000000002));
#369337=CARTESIAN_POINT('Origin',(1.38777878078145E-16,1.38777878078145E-16,
-4.19687500000002));
#369338=CARTESIAN_POINT('',(2.14914986703435E-17,-0.957716426222737,-3.10000000000001));
#369339=CARTESIAN_POINT('',(2.14915015512999E-17,-0.957716426222737,-3.04375000000002));
#369340=CARTESIAN_POINT('',(1.60269320569837E-16,-0.957716426222737,-4.19687500000002));
#369341=CARTESIAN_POINT('Ctrl Pts',(-1.17286435586452E-16,-0.957716426222737,
-3.10000000000001));
#369342=CARTESIAN_POINT('Ctrl Pts',(0.552937836487023,-0.957716426222737,
-3.06250000000001));
#369343=CARTESIAN_POINT('Ctrl Pts',(0.829406754730535,-0.478858213111369,
-3.02500000000001));
#369344=CARTESIAN_POINT('Ctrl Pts',(1.10587567297405,-3.36181115481189E-16,
-2.98750000000001));
#369345=CARTESIAN_POINT('Ctrl Pts',(0.829406754730536,0.478858213111368,
-2.95000000000001));
#369346=CARTESIAN_POINT('Ctrl Pts',(0.552937836487024,0.957716426222737,
-2.91250000000001));
#369347=CARTESIAN_POINT('Ctrl Pts',(0.,0.957716426222737,-2.87500000000001));
#369348=CARTESIAN_POINT('Ctrl Pts',(-0.552937836487023,0.957716426222737,
-2.83750000000001));
#369349=CARTESIAN_POINT('Ctrl Pts',(-0.829406754730535,0.478858213111368,
-2.80000000000001));
#369350=CARTESIAN_POINT('Ctrl Pts',(-1.10587567297405,-6.51183955268371E-17,
-2.76250000000001));
#369351=CARTESIAN_POINT('Ctrl Pts',(-0.829406754730535,-0.478858213111368,
-2.72500000000001));
#369352=CARTESIAN_POINT('Ctrl Pts',(-0.552937836487024,-0.957716426222737,
-2.68750000000001));
#369353=CARTESIAN_POINT('Ctrl Pts',(-1.17286435586452E-16,-0.957716426222737,
-2.65000000000001));
#369354=CARTESIAN_POINT('Ctrl Pts',(-1.17286435586452E-16,-0.957716426222737,
-3.04375000000002));
#369355=CARTESIAN_POINT('Ctrl Pts',(0.552937836487023,-0.957716426222737,
-3.00625000000002));
#369356=CARTESIAN_POINT('Ctrl Pts',(0.829406754730535,-0.478858213111369,
-2.96875000000002));
#369357=CARTESIAN_POINT('Ctrl Pts',(1.10587567297405,-3.3613079065073E-16,
-2.93125000000002));
#369358=CARTESIAN_POINT('Ctrl Pts',(0.829406754730536,0.478858213111368,
-2.89375000000002));
#369359=CARTESIAN_POINT('Ctrl Pts',(0.552937836487024,0.957716426222737,
-2.85625000000002));
#369360=CARTESIAN_POINT('Ctrl Pts',(0.,0.957716426222737,-2.81875000000002));
#369361=CARTESIAN_POINT('Ctrl Pts',(-0.552937836487023,0.957716426222737,
-2.78125000000002));
#369362=CARTESIAN_POINT('Ctrl Pts',(-0.829406754730535,0.478858213111368,
-2.74375000000002));
#369363=CARTESIAN_POINT('Ctrl Pts',(-1.10587567297405,-6.50680706963789E-17,
-2.70625000000002));
#369364=CARTESIAN_POINT('Ctrl Pts',(-0.829406754730535,-0.478858213111368,
-2.66875000000002));
#369365=CARTESIAN_POINT('Ctrl Pts',(-0.552937836487024,-0.957716426222737,
-2.63125000000002));
#369366=CARTESIAN_POINT('Ctrl Pts',(-1.17286435586452E-16,-0.957716426222737,
-2.59375000000002));
#369367=CARTESIAN_POINT('Origin',(1.38777878078145E-16,1.38777878078145E-16,
-4.19687500000002));
#369368=CARTESIAN_POINT('',(2.1491475622692E-17,-0.957716426222737,-3.55000000000001));
#369369=CARTESIAN_POINT('',(2.14914785036484E-17,-0.957716426222737,-3.49375000000002));
#369370=CARTESIAN_POINT('',(1.60269320569837E-16,-0.957716426222737,-4.19687500000002));
#369371=CARTESIAN_POINT('Ctrl Pts',(-1.17286435586452E-16,-0.957716426222737,
-3.55000000000001));
#369372=CARTESIAN_POINT('Ctrl Pts',(0.552937836487023,-0.957716426222737,
-3.51250000000001));
#369373=CARTESIAN_POINT('Ctrl Pts',(0.829406754730535,-0.478858213111369,
-3.47500000000001));
#369374=CARTESIAN_POINT('Ctrl Pts',(1.10587567297405,-3.36583714124855E-16,
-3.43750000000001));
#369375=CARTESIAN_POINT('Ctrl Pts',(0.829406754730536,0.478858213111368,
-3.40000000000001));
#369376=CARTESIAN_POINT('Ctrl Pts',(0.552937836487024,0.957716426222737,
-3.36250000000001));
#369377=CARTESIAN_POINT('Ctrl Pts',(0.,0.957716426222737,-3.32500000000001));
#369378=CARTESIAN_POINT('Ctrl Pts',(-0.552937836487023,0.957716426222737,
-3.28750000000001));
#369379=CARTESIAN_POINT('Ctrl Pts',(-0.829406754730535,0.478858213111368,
-3.25000000000001));
#369380=CARTESIAN_POINT('Ctrl Pts',(-1.10587567297405,-6.55209941705032E-17,
-3.21250000000001));
#369381=CARTESIAN_POINT('Ctrl Pts',(-0.829406754730535,-0.478858213111368,
-3.17500000000001));
#369382=CARTESIAN_POINT('Ctrl Pts',(-0.552937836487024,-0.957716426222737,
-3.13750000000001));
#369383=CARTESIAN_POINT('Ctrl Pts',(-1.17286435586452E-16,-0.957716426222737,
-3.10000000000001));
#369384=CARTESIAN_POINT('Ctrl Pts',(-1.17286435586452E-16,-0.957716426222737,
-3.49375000000002));
#369385=CARTESIAN_POINT('Ctrl Pts',(0.552937836487023,-0.957716426222737,
-3.45625000000002));
#369386=CARTESIAN_POINT('Ctrl Pts',(0.829406754730535,-0.478858213111369,
-3.41875000000002));
#369387=CARTESIAN_POINT('Ctrl Pts',(1.10587567297405,-3.36533389294396E-16,
-3.38125000000002));
#369388=CARTESIAN_POINT('Ctrl Pts',(0.829406754730536,0.478858213111368,
-3.34375000000002));
#369389=CARTESIAN_POINT('Ctrl Pts',(0.552937836487024,0.957716426222737,
-3.30625000000002));
#369390=CARTESIAN_POINT('Ctrl Pts',(0.,0.957716426222737,-3.26875000000002));
#369391=CARTESIAN_POINT('Ctrl Pts',(-0.552937836487023,0.957716426222737,
-3.23125000000002));
#369392=CARTESIAN_POINT('Ctrl Pts',(-0.829406754730535,0.478858213111368,
-3.19375000000002));
#369393=CARTESIAN_POINT('Ctrl Pts',(-1.10587567297405,-6.54706693400449E-17,
-3.15625000000002));
#369394=CARTESIAN_POINT('Ctrl Pts',(-0.829406754730535,-0.478858213111368,
-3.11875000000002));
#369395=CARTESIAN_POINT('Ctrl Pts',(-0.552937836487024,-0.957716426222737,
-3.08125000000002));
#369396=CARTESIAN_POINT('Ctrl Pts',(-1.17286435586452E-16,-0.957716426222737,
-3.04375000000002));
#369397=CARTESIAN_POINT('Origin',(1.38777878078145E-16,1.38777878078145E-16,
-4.19687500000002));
#369398=CARTESIAN_POINT('',(1.60269345368232E-16,-0.957716426222737,-3.95478357377733));
#369399=CARTESIAN_POINT('',(2.14914554559969E-17,-0.957716426222737,-3.94375000000002));
#369400=CARTESIAN_POINT('',(1.60269320569837E-16,-0.957716426222737,-4.19687500000002));
#369401=CARTESIAN_POINT('',(0.561651082536657,-0.775737593869378,-3.95478357377714));
#369402=CARTESIAN_POINT('Origin',(-4.58730275987307E-13,1.7608137170555E-12,
-3.95478357377551));
#369403=CARTESIAN_POINT('Ctrl Pts',(0.561651082536657,-0.775737593869378,
-3.95478357377714));
#369404=CARTESIAN_POINT('Ctrl Pts',(0.727208897839709,-0.655870093670933,
-3.93886202708702));
#369405=CARTESIAN_POINT('Ctrl Pts',(0.829406754730535,-0.478858213111369,
-3.92500000000001));
#369406=CARTESIAN_POINT('Ctrl Pts',(1.10587567297405,-3.36986312768521E-16,
-3.88750000000001));
#369407=CARTESIAN_POINT('Ctrl Pts',(0.829406754730536,0.478858213111368,
-3.85000000000001));
#369408=CARTESIAN_POINT('Ctrl Pts',(0.552937836487024,0.957716426222737,
-3.81250000000001));
#369409=CARTESIAN_POINT('Ctrl Pts',(0.,0.957716426222737,-3.77500000000001));
#369410=CARTESIAN_POINT('Ctrl Pts',(-0.552937836487023,0.957716426222737,
-3.73750000000001));
#369411=CARTESIAN_POINT('Ctrl Pts',(-0.829406754730535,0.478858213111368,
-3.70000000000001));
#369412=CARTESIAN_POINT('Ctrl Pts',(-1.10587567297405,-6.59235928141692E-17,
-3.66250000000001));
#369413=CARTESIAN_POINT('Ctrl Pts',(-0.829406754730535,-0.478858213111368,
-3.62500000000001));
#369414=CARTESIAN_POINT('Ctrl Pts',(-0.552937836487024,-0.957716426222737,
-3.58750000000001));
#369415=CARTESIAN_POINT('Ctrl Pts',(-1.17286435586452E-16,-0.957716426222737,
-3.55000000000001));
#369416=CARTESIAN_POINT('Ctrl Pts',(-1.17286435586452E-16,-0.957716426222737,
-3.94375000000002));
#369417=CARTESIAN_POINT('Ctrl Pts',(0.552937836487023,-0.957716426222737,
-3.90625000000002));
#369418=CARTESIAN_POINT('Ctrl Pts',(0.829406754730535,-0.478858213111369,
-3.86875000000002));
#369419=CARTESIAN_POINT('Ctrl Pts',(1.10587567297405,-3.36935987938062E-16,
-3.83125000000002));
#369420=CARTESIAN_POINT('Ctrl Pts',(0.829406754730536,0.478858213111368,
-3.79375000000002));
#369421=CARTESIAN_POINT('Ctrl Pts',(0.552937836487024,0.957716426222737,
-3.75625000000002));
#369422=CARTESIAN_POINT('Ctrl Pts',(0.,0.957716426222737,-3.71875000000002));
#369423=CARTESIAN_POINT('Ctrl Pts',(-0.552937836487023,0.957716426222737,
-3.68125000000002));
#369424=CARTESIAN_POINT('Ctrl Pts',(-0.829406754730535,0.478858213111368,
-3.64375000000002));
#369425=CARTESIAN_POINT('Ctrl Pts',(-1.10587567297405,-6.58732679837109E-17,
-3.60625000000002));
#369426=CARTESIAN_POINT('Ctrl Pts',(-0.829406754730535,-0.478858213111368,
-3.56875000000002));
#369427=CARTESIAN_POINT('Ctrl Pts',(-0.552937836487024,-0.957716426222737,
-3.53125000000002));
#369428=CARTESIAN_POINT('Ctrl Pts',(-1.17286435586452E-16,-0.957716426222737,
-3.49375000000002));
#369429=CARTESIAN_POINT('Origin',(0.,0.,2.95));
#369430=CARTESIAN_POINT('',(5.80020015507564E-14,1.25000000000001,-3.49375000000003));
#369431=CARTESIAN_POINT('',(7.48635137372505E-14,1.25000000000001,-3.55000000000002));
#369432=CARTESIAN_POINT('',(-1.5308084989342E-16,1.25000000000001,2.95));
#369433=CARTESIAN_POINT('',(0.875786586618201,-0.891906864366224,-3.66249999999728));
#369434=CARTESIAN_POINT('Ctrl Pts',(1.16157083951406E-13,1.25000000000001,
-3.49375000000003));
#369435=CARTESIAN_POINT('Ctrl Pts',(0.0558262619039152,1.25000000000001,
-3.49665081766045));
#369436=CARTESIAN_POINT('Ctrl Pts',(0.111699054709194,1.24626059886401,
-3.49966623517157));
#369437=CARTESIAN_POINT('Ctrl Pts',(0.333022130666348,1.2163788867422,-3.51206297090858));
#369438=CARTESIAN_POINT('Ctrl Pts',(0.492605203231851,1.16095117575365,
-3.52201798192958));
#369439=CARTESIAN_POINT('Ctrl Pts',(0.774960304797056,0.993884904164799,
-3.54170157152786));
#369440=CARTESIAN_POINT('Ctrl Pts',(0.896304252028742,0.886014998629642,
-3.5512428851478));
#369441=CARTESIAN_POINT('Ctrl Pts',(1.09217035418525,0.62923090622271,-3.56912390913247));
#369442=CARTESIAN_POINT('Ctrl Pts',(1.16446017056606,0.482499223607466,
-3.57730004658363));
#369443=CARTESIAN_POINT('Ctrl Pts',(1.2498202949631,0.166545811296484,-3.59625725132228));
#369444=CARTESIAN_POINT('Ctrl Pts',(1.26086616979021,0.000109175634494391,
-3.606243449462));
#369445=CARTESIAN_POINT('Ctrl Pts',(1.22094386548057,-0.302209608995765,
-3.62438257653982));
#369446=CARTESIAN_POINT('Ctrl Pts',(1.17953231039141,-0.436750102582941,
-3.63245500615505));
#369447=CARTESIAN_POINT('Ctrl Pts',(1.05507856256371,-0.684196471505689,
-3.64730178829041));
#369448=CARTESIAN_POINT('Ctrl Pts',(0.973700164305609,-0.795762971529037,
-3.65452794446843));
#369449=CARTESIAN_POINT('Ctrl Pts',(0.875786586616994,-0.891906864365204,
-3.66249999999274));
#369450=CARTESIAN_POINT('',(1.25000000000001,1.00721982129472E-13,-3.6625));
#369451=CARTESIAN_POINT('Origin',(0.,-9.76875228502569E-17,-3.6625));
#369452=CARTESIAN_POINT('Ctrl Pts',(1.25000000000001,-1.72868663828041E-12,
-3.66250000000011));
#369453=CARTESIAN_POINT('Ctrl Pts',(1.25000000000022,0.154429265794931,
-3.65323424405232));
#369454=CARTESIAN_POINT('Ctrl Pts',(1.22138437816133,0.307537553418373,
-3.64404774679489));
#369455=CARTESIAN_POINT('Ctrl Pts',(1.11179970332925,0.590395200419514,
-3.62707628797482));
#369456=CARTESIAN_POINT('Ctrl Pts',(1.03366513337583,0.718472897613953,
-3.61965662894215));
#369457=CARTESIAN_POINT('Ctrl Pts',(0.827234960889385,0.951025440084063,
-3.6019536262592));
#369458=CARTESIAN_POINT('Ctrl Pts',(0.697099868255548,1.05014772137054,
-3.59221794005192));
#369459=CARTESIAN_POINT('Ctrl Pts',(0.402996178943989,1.19480263661878,
-3.57259621661704));
#369460=CARTESIAN_POINT('Ctrl Pts',(0.241205989437471,1.23765799933533,
-3.5629036908838));
#369461=CARTESIAN_POINT('Ctrl Pts',(0.0504979547264238,1.2492356898471,
-3.55264688000252));
#369462=CARTESIAN_POINT('Ctrl Pts',(0.0252376533412523,1.25000000000001,
-3.55131138693554));
#369463=CARTESIAN_POINT('Ctrl Pts',(1.49880108324394E-13,1.25000000000001,
-3.55000000000002));
#369464=CARTESIAN_POINT('Origin',(0.,0.,2.95));
#369465=CARTESIAN_POINT('',(-7.654042494671E-17,1.25000000000001,-3.04375000000002));
#369466=CARTESIAN_POINT('',(1.01092532694019E-13,1.25000000000001,-3.10000000000002));
#369467=CARTESIAN_POINT('',(-1.5308084989342E-16,1.25000000000001,2.95));
#369468=CARTESIAN_POINT('Ctrl Pts',(0.,1.25000000000001,-3.04375000000002));
#369469=CARTESIAN_POINT('Ctrl Pts',(0.0801005201788763,1.25000000000001,
-3.0479121451199));
#369470=CARTESIAN_POINT('Ctrl Pts',(0.160186539952716,1.24230243878038,
-3.05230446361325));
#369471=CARTESIAN_POINT('Ctrl Pts',(0.40239322377935,1.19508772134168,-3.06630633360603));
#369472=CARTESIAN_POINT('Ctrl Pts',(0.557624581099529,1.13101732560779,
-3.07629450341224));
#369473=CARTESIAN_POINT('Ctrl Pts',(0.828663890971705,0.949425856712451,
-3.09582586314551));
#369474=CARTESIAN_POINT('Ctrl Pts',(0.943270166994007,0.83567394848635,
-3.1051935371804));
#369475=CARTESIAN_POINT('Ctrl Pts',(1.12600178305657,0.567228567228114,
-3.12274191191323));
#369476=CARTESIAN_POINT('Ctrl Pts',(1.19087205499603,0.414087629904788,
-3.13140474220578));
#369477=CARTESIAN_POINT('Ctrl Pts',(1.25738607605826,0.0919088285462163,
-3.15073547028729));
#369478=CARTESIAN_POINT('Ctrl Pts',(1.25857313222639,-0.0738927601021803,
-3.16068356560619));
#369479=CARTESIAN_POINT('Ctrl Pts',(1.19787636075818,-0.390746558040131,
-3.17969479348247));
#369480=CARTESIAN_POINT('Ctrl Pts',(1.13878777518423,-0.539192113889463,
-3.18825261484703));
#369481=CARTESIAN_POINT('Ctrl Pts',(0.964401571050862,-0.812343959042414,
-3.20550854317256));
#369482=CARTESIAN_POINT('Ctrl Pts',(0.84832420071093,-0.932898580437442,
-3.21515673890554));
#369483=CARTESIAN_POINT('Ctrl Pts',(0.578771305933263,-1.11976065620169,
-3.23476898045094));
#369484=CARTESIAN_POINT('Ctrl Pts',(0.428640235704609,-1.1853755909506,
-3.24453846773632));
#369485=CARTESIAN_POINT('Ctrl Pts',(0.114671973971978,-1.25487465779539,
-3.26293770918022));
#369486=CARTESIAN_POINT('Ctrl Pts',(-0.0459245874231769,-1.2592653387857,
-3.27085835139851));
#369487=CARTESIAN_POINT('Ctrl Pts',(-0.367625069297885,-1.20630429357242,
-3.2891632301377));
#369488=CARTESIAN_POINT('Ctrl Pts',(-0.525104066239286,-1.1465479638438,
-3.29913876874438));
#369489=CARTESIAN_POINT('Ctrl Pts',(-0.801932878622589,-0.972181167374948,
-3.31875421967985));
#369490=CARTESIAN_POINT('Ctrl Pts',(-0.919967305363899,-0.861340512618317,
-3.32821268804729));
#369491=CARTESIAN_POINT('Ctrl Pts',(-1.10934819693316,-0.598757638681498,
-3.34593069405082));
#369492=CARTESIAN_POINT('Ctrl Pts',(-1.17799385288076,-0.44889238620976,
-3.35431645682749));
#369493=CARTESIAN_POINT('Ctrl Pts',(-1.25410425134268,-0.129813702317056,
-3.37346117786105));
#369494=CARTESIAN_POINT('Ctrl Pts',(-1.2602788701469,0.0363811147974186,
-3.38343286688791));
#369495=CARTESIAN_POINT('Ctrl Pts',(-1.20880266299188,0.355630032051346,
-3.40258780192315));
#369496=CARTESIAN_POINT('Ctrl Pts',(-1.15395901910286,0.505981224656806,
-3.41146796721162));
#369497=CARTESIAN_POINT('Ctrl Pts',(-0.987406810821905,0.784214035498693,
-3.42846925814254));
#369498=CARTESIAN_POINT('Ctrl Pts',(-0.874873756978497,0.908041106904038,
-3.43803145928833));
#369499=CARTESIAN_POINT('Ctrl Pts',(-0.610488461751786,1.10285608983475,
-3.45761377169945));
#369500=CARTESIAN_POINT('Ctrl Pts',(-0.461856329770814,1.17289478537514,
-3.46743808469252));
#369501=CARTESIAN_POINT('Ctrl Pts',(-0.204354382331899,1.23745189198145,
-3.48275499157107));
#369502=CARTESIAN_POINT('Ctrl Pts',(-0.102275013815502,1.25000000000001,
-3.48843563439182));
#369503=CARTESIAN_POINT('Ctrl Pts',(1.16209125655686E-13,1.25000000000001,
-3.49375000000003));
#369504=CARTESIAN_POINT('Ctrl Pts',(1.49984191732955E-13,1.25000000000001,
-3.55000000000002));
#369505=CARTESIAN_POINT('Ctrl Pts',(-0.132674294559962,1.25000000000001,
-3.54310604142893));
#369506=CARTESIAN_POINT('Ctrl Pts',(-0.26465747431644,1.228882811502,-3.53561447858149));
#369507=CARTESIAN_POINT('Ctrl Pts',(-0.546731051132629,1.13598604793516,
-3.51817060267893));
#369508=CARTESIAN_POINT('Ctrl Pts',(-0.690850975295588,1.05456313893759,
-3.50823922447801));
#369509=CARTESIAN_POINT('Ctrl Pts',(-0.940700856621858,0.839649471497178,
-3.48880923379313));
#369510=CARTESIAN_POINT('Ctrl Pts',(-1.04351636963,0.707800398739344,-3.47996802392435));
#369511=CARTESIAN_POINT('Ctrl Pts',(-1.18921447801218,0.416897828238739,
-3.46251386969432));
#369512=CARTESIAN_POINT('Ctrl Pts',(-1.23270515879014,0.261640644464715,
-3.45319843866788));
#369513=CARTESIAN_POINT('Ctrl Pts',(-1.25939974289888,-0.0630143527908859,
-3.43371913883254));
#369514=CARTESIAN_POINT('Ctrl Pts',(-1.23991046724957,-0.229540855795417,
-3.42372754865227));
#369515=CARTESIAN_POINT('Ctrl Pts',(-1.13875725577918,-0.539856394523013,
-3.40510861632861));
#369516=CARTESIAN_POINT('Ctrl Pts',(-1.06020700578772,-0.681302486930842,
-3.39715089740901));
#369517=CARTESIAN_POINT('Ctrl Pts',(-0.85308723432579,-0.927829827179376,
-3.37899281817883));
#369518=CARTESIAN_POINT('Ctrl Pts',(-0.726101406925719,-1.03023901135182,
-3.36932216550672));
#369519=CARTESIAN_POINT('Ctrl Pts',(-0.436568842699685,-1.18295211451495,
-3.34969621906127));
#369520=CARTESIAN_POINT('Ctrl Pts',(-0.276028747136534,-1.23036286746581,
-3.33993198840772));
#369521=CARTESIAN_POINT('Ctrl Pts',(0.0467989359121036,-1.25911687906126,
-3.32229474958596));
#369522=CARTESIAN_POINT('Ctrl Pts',(0.205727709267049,-1.2430821436253,
-3.3141025389595));
#369523=CARTESIAN_POINT('Ctrl Pts',(0.51413235956892,-1.15104145573479,
-3.29531614261438));
#369524=CARTESIAN_POINT('Ctrl Pts',(0.66010527760148,-1.07400506479895,
-3.28542007556946));
#369525=CARTESIAN_POINT('Ctrl Pts',(0.917020015673747,-0.865760355830752,
-3.26582305291378));
#369526=CARTESIAN_POINT('Ctrl Pts',(1.02444705071578,-0.73548782844564,
-3.25662926970673));
#369527=CARTESIAN_POINT('Ctrl Pts',(1.1780467288341,-0.44733973729301,-3.23934038423758));
#369528=CARTESIAN_POINT('Ctrl Pts',(1.22542020036252,-0.293656149941834,
-3.23011936899651));
#369529=CARTESIAN_POINT('Ctrl Pts',(1.26057525901858,0.0293356889581505,
-3.21073985866251));
#369530=CARTESIAN_POINT('Ctrl Pts',(1.24561377045063,0.195865703788074,
-3.20074805777271));
#369531=CARTESIAN_POINT('Ctrl Pts',(1.15289542449753,0.509239004921235,
-3.18194565970473));
#369532=CARTESIAN_POINT('Ctrl Pts',(1.07769691096265,0.653497200184776,
-3.17389385814288));
#369533=CARTESIAN_POINT('Ctrl Pts',(0.876616464365373,0.905559960847434,
-3.15588352882554));
#369534=CARTESIAN_POINT('Ctrl Pts',(0.752640825960971,1.01094764575026,
-3.14627993513994));
#369535=CARTESIAN_POINT('Ctrl Pts',(0.46757179903791,1.17104730599246,-3.12666432418383));
#369536=CARTESIAN_POINT('Ctrl Pts',(0.308316758016824,1.22267363848955,
-3.11684039953662));
#369537=CARTESIAN_POINT('Ctrl Pts',(0.0958504907300428,1.24724676713127,
-3.10506313458231));
#369538=CARTESIAN_POINT('Ctrl Pts',(0.0479017666976706,1.25000000000001,
-3.10248904881079));
#369539=CARTESIAN_POINT('Ctrl Pts',(2.02338146237931E-13,1.25000000000001,
-3.10000000000002));
#369540=CARTESIAN_POINT('Origin',(0.,0.,2.95));
#369541=CARTESIAN_POINT('',(-7.12695918790362E-14,1.25000000000001,-2.59375000000002));
#369542=CARTESIAN_POINT('',(1.79696092910825E-15,1.25000000000001,-2.65000000000001));
#369543=CARTESIAN_POINT('',(-1.5308084989342E-16,1.25000000000001,2.95));
#369544=CARTESIAN_POINT('Ctrl Pts',(-1.42386102908176E-13,1.25000000000001,
-2.59375000000002));
#369545=CARTESIAN_POINT('Ctrl Pts',(0.105342329382033,1.25000000000002,
-2.59922374800034));
#369546=CARTESIAN_POINT('Ctrl Pts',(0.210464993290618,1.23668796757782,
-2.60508544282054));
#369547=CARTESIAN_POINT('Ctrl Pts',(0.472931271974733,1.16882871805381,
-2.62075936820489));
#369548=CARTESIAN_POINT('Ctrl Pts',(0.623176125175293,1.09611624799401,
-2.63074769388626));
#369549=CARTESIAN_POINT('Ctrl Pts',(0.881712267495814,0.900217730807902,
-2.6500585814246));
#369550=CARTESIAN_POINT('Ctrl Pts',(0.989034488987936,0.78079342394926,
-2.65921793684252));
#369551=CARTESIAN_POINT('Ctrl Pts',(1.15647945686897,0.502488376758182,
-2.67626778401351));
#369552=CARTESIAN_POINT('Ctrl Pts',(1.21284945899906,0.344928507153231,
-2.68555428957086));
#369553=CARTESIAN_POINT('Ctrl Pts',(1.2604713269282,0.019338514041045,-2.70508968915759));
#369554=CARTESIAN_POINT('Ctrl Pts',(1.2522183870622,-0.145308449334908,
-2.71496850696015));
#369555=CARTESIAN_POINT('Ctrl Pts',(1.17405124976896,-0.457385009487385,
-2.73369310056929));
#369556=CARTESIAN_POINT('Ctrl Pts',(1.10671349811452,-0.602306727205998,
-2.74181268157154));
#369557=CARTESIAN_POINT('Ctrl Pts',(0.917179620939207,-0.86531427570947,
-2.75955137717734));
#369558=CARTESIAN_POINT('Ctrl Pts',(0.794466491816304,-0.979180490624983,
-2.7693437248567));
#369559=CARTESIAN_POINT('Ctrl Pts',(0.515519595225215,-1.15012812765669,
-2.78896665989293));
#369560=CARTESIAN_POINT('Ctrl Pts',(0.362833793640631,-1.20702852828054,
-2.79860745888981));
#369561=CARTESIAN_POINT('Ctrl Pts',(0.0449590270720812,-1.25948835649622,
-2.81669851112051));
#369562=CARTESIAN_POINT('Ctrl Pts',(-0.117152741739399,-1.25483438374123,
-2.82469240351598));
#369563=CARTESIAN_POINT('Ctrl Pts',(-0.435769191696286,-1.18325981368898,
-2.84339543700112));
#369564=CARTESIAN_POINT('Ctrl Pts',(-0.588713704895264,-1.1150817006434,
-2.85338801042048));
#369565=CARTESIAN_POINT('Ctrl Pts',(-0.853965955173471,-0.926661281286531,
-2.8728235342303));
#369566=CARTESIAN_POINT('Ctrl Pts',(-0.965181724295405,-0.810185693519208,
-2.88209674274498));
#369567=CARTESIAN_POINT('Ctrl Pts',(-1.1413894115652,-0.536069156456338,
-2.89947625886793));
#369568=CARTESIAN_POINT('Ctrl Pts',(-1.20250854929645,-0.379656750626062,
-2.9084705949625));
#369569=CARTESIAN_POINT('Ctrl Pts',(-1.25949740328438,-0.0545476131985929,
-2.92797714320814));
#369570=CARTESIAN_POINT('Ctrl Pts',(-1.25580678653293,0.110725047297354,
-2.9378935028379));
#369571=CARTESIAN_POINT('Ctrl Pts',(-1.18609130510389,0.425150928291168,
-2.95675905569753));
#369572=CARTESIAN_POINT('Ctrl Pts',(-1.12278089789272,0.571763500175269,
-2.96506149817778));
#369573=CARTESIAN_POINT('Ctrl Pts',(-0.94062407355898,0.839766230910028,
-2.98256672634057));
#369574=CARTESIAN_POINT('Ctrl Pts',(-0.821104779434934,0.956948443351132,
-2.99229259741103));
#369575=CARTESIAN_POINT('Ctrl Pts',(-0.546631107919309,1.13573250749033,
-3.01191818966735));
#369576=CARTESIAN_POINT('Ctrl Pts',(-0.39513175643769,1.19690191271148,
-3.02162540904638));
#369577=CARTESIAN_POINT('Ctrl Pts',(-0.158157705063089,1.242496613601,-3.03530678298476));
#369578=CARTESIAN_POINT('Ctrl Pts',(-0.0790836106868099,1.25000000000001,
-3.03964069504736));
#369579=CARTESIAN_POINT('Ctrl Pts',(0.,1.25000000000001,-3.04375000000002));
#369580=CARTESIAN_POINT('Ctrl Pts',(1.98504407356026E-13,1.25000000000001,
-3.10000000000002));
#369581=CARTESIAN_POINT('Ctrl Pts',(-0.110023330863273,1.25000000000001,
-3.09428302002783));
#369582=CARTESIAN_POINT('Ctrl Pts',(-0.219753373684046,1.23547878878256,
-3.08814564341281));
#369583=CARTESIAN_POINT('Ctrl Pts',(-0.483784337213042,1.16406351081363,
-3.07228373376564));
#369584=CARTESIAN_POINT('Ctrl Pts',(-0.631346657530357,1.09109489844724,
-3.06242711231248));
#369585=CARTESIAN_POINT('Ctrl Pts',(-0.892250491426103,0.890989610552251,
-3.04286699278972));
#369586=CARTESIAN_POINT('Ctrl Pts',(-1.00234506247223,0.76500253803068,
-3.03340015228184));
#369587=CARTESIAN_POINT('Ctrl Pts',(-1.1636454044465,0.483408458576927,
-3.01650450751462));
#369588=CARTESIAN_POINT('Ctrl Pts',(-1.21560102978879,0.331735897822884,
-3.00740415386937));
#369589=CARTESIAN_POINT('Ctrl Pts',(-1.26079895223703,0.0110195436563138,
-2.98816117261938));
#369590=CARTESIAN_POINT('Ctrl Pts',(-1.25124075256951,-0.155358063370983,
-2.97817851619774));
#369591=CARTESIAN_POINT('Ctrl Pts',(-1.16869360067347,-0.472275959171684,
-2.9591634424497));
#369592=CARTESIAN_POINT('Ctrl Pts',(-1.09751310445712,-0.619957886750929,
-2.95092971716425));
#369593=CARTESIAN_POINT('Ctrl Pts',(-0.903627337233052,-0.878521253299362,
-2.9330982161769));
#369594=CARTESIAN_POINT('Ctrl Pts',(-0.783289989381195,-0.987312035831273,
-2.92358158068511));
#369595=CARTESIAN_POINT('Ctrl Pts',(-0.502608934507082,-1.15663399822554,
-2.90391730638037));
#369596=CARTESIAN_POINT('Ctrl Pts',(-0.343658713220788,-1.2133959834479,
-2.89395515104943));
#369597=CARTESIAN_POINT('Ctrl Pts',(-0.0209816289176561,-1.25988228237505,
-2.87579376894808));
#369598=CARTESIAN_POINT('Ctrl Pts',(0.13913046002791,-1.25235370103634,
-2.86784118026163));
#369599=CARTESIAN_POINT('Ctrl Pts',(0.451659987362524,-1.17683970593185,
-2.84933624980222));
#369600=CARTESIAN_POINT('Ctrl Pts',(0.600767646557596,-1.10816080217134,
-2.8395280214437));
#369601=CARTESIAN_POINT('Ctrl Pts',(0.866770480060013,-0.915781193785182,
-2.81993472051462));
#369602=CARTESIAN_POINT('Ctrl Pts',(0.980405780280576,-0.792951045382059,
-2.81034515265706));
#369603=CARTESIAN_POINT('Ctrl Pts',(1.14937757073535,-0.516276107469031,
-2.79326487273626));
#369604=CARTESIAN_POINT('Ctrl Pts',(1.20553169019293,-0.366519856087064,
-2.78449119136523));
#369605=CARTESIAN_POINT('Ctrl Pts',(1.25986993086269,-0.0480047442141254,
-2.76538028465285));
#369606=CARTESIAN_POINT('Ctrl Pts',(1.25524295575607,0.118083896291753,
-2.7554149662225));
#369607=CARTESIAN_POINT('Ctrl Pts',(1.18209588403663,0.438135514494601,
-2.73621186913033));
#369608=CARTESIAN_POINT('Ctrl Pts',(1.11461619357743,0.589009815920291,
-2.72774686186885));
#369609=CARTESIAN_POINT('Ctrl Pts',(0.927297001734213,0.853419375895082,
-2.71008118434445));
#369610=CARTESIAN_POINT('Ctrl Pts',(0.810322094209521,0.965177306505159,
-2.70065025193484));
#369611=CARTESIAN_POINT('Ctrl Pts',(0.535275736301416,1.14181259951419,
-2.68105936515457));
#369612=CARTESIAN_POINT('Ctrl Pts',(0.378484215519997,1.20292015139326,
-2.67107901219251));
#369613=CARTESIAN_POINT('Ctrl Pts',(0.14337927547669,1.24383556877028,-2.65763513863324));
#369614=CARTESIAN_POINT('Ctrl Pts',(0.0716801446618524,1.25000000000001,
-2.65372460957346));
#369615=CARTESIAN_POINT('Ctrl Pts',(3.74700270810992E-15,1.25000000000001,
-2.65000000000001));
#369616=CARTESIAN_POINT('Origin',(0.,0.,2.95));
#369617=CARTESIAN_POINT('',(-1.34968637916908E-13,1.25000000000001,-2.14375000000001));
#369618=CARTESIAN_POINT('',(-2.06850553195514E-14,1.25000000000001,-2.20000000000001));
#369619=CARTESIAN_POINT('',(-1.5308084989342E-16,1.25000000000001,2.95));
#369620=CARTESIAN_POINT('Ctrl Pts',(-2.70200528618147E-13,1.25000000000001,
-2.14375000000001));
#369621=CARTESIAN_POINT('Ctrl Pts',(0.130400599680054,1.25000000000003,
-2.15052581391952));
#369622=CARTESIAN_POINT('Ctrl Pts',(0.260188488106204,1.22960103321381,
-2.15788175943196));
#369623=CARTESIAN_POINT('Ctrl Pts',(0.541027657753502,1.13876865933085,
-2.17519956196599));
#369624=CARTESIAN_POINT('Ctrl Pts',(0.6858869727539,1.0578577579882,-2.18515399981218));
#369625=CARTESIAN_POINT('Ctrl Pts',(0.931518979784196,0.848456115260838,
-2.20419946257825));
#369626=CARTESIAN_POINT('Ctrl Pts',(1.03141898990211,0.723707518137767,
-2.21282754891178));
#369627=CARTESIAN_POINT('Ctrl Pts',(1.18275495824577,0.437106100705102,
-2.23002363395774));
#369628=CARTESIAN_POINT('Ctrl Pts',(1.23021426454136,0.276629885961306,
-2.23965220684237));
#369629=CARTESIAN_POINT('Ctrl Pts',(1.25950792098496,-0.0501476581208609,
-2.2592588594873));
#369630=CARTESIAN_POINT('Ctrl Pts',(1.24234770403752,-0.21320020716703,
-2.26904201243007));
#369631=CARTESIAN_POINT('Ctrl Pts',(1.14757966301889,-0.520460564018815,
-2.28747763384117));
#369632=CARTESIAN_POINT('Ctrl Pts',(1.07210138549065,-0.662128816518621,
-2.29540584237956));
#369633=CARTESIAN_POINT('Ctrl Pts',(0.867140045341389,-0.91565552203857,
-2.31366174718694));
#369634=CARTESIAN_POINT('Ctrl Pts',(0.737281518839768,-1.02311320506751,
-2.32363312464871));
#369635=CARTESIAN_POINT('Ctrl Pts',(0.448686870271631,-1.1776864945793,
-2.34326614115744));
#369636=CARTESIAN_POINT('Ctrl Pts',(0.293886489933415,-1.22552458722037,
-2.35274494764997));
#369637=CARTESIAN_POINT('Ctrl Pts',(-0.0277882329935411,-1.26027459942359,
-2.37050215692467));
#369638=CARTESIAN_POINT('Ctrl Pts',(-0.191681604333076,-1.24592573976443,
-2.37883229613455));
#369639=CARTESIAN_POINT('Ctrl Pts',(-0.50653836891461,-1.15459340299165,
-2.39793270363859));
#369640=CARTESIAN_POINT('Ctrl Pts',(-0.654198020566734,-1.07781669916157,
-2.40790862532018));
#369641=CARTESIAN_POINT('Ctrl Pts',(-0.906488342174939,-0.875205244858828,
-2.42709635860776));
#369642=CARTESIAN_POINT('Ctrl Pts',(-1.01015543604116,-0.753159657325788,
-2.4360604205605));
#369643=CARTESIAN_POINT('Ctrl Pts',(-1.16974926270548,-0.470795286726956,
-2.45300228279643));
#369644=CARTESIAN_POINT('Ctrl Pts',(-1.22177589738895,-0.311775055933201,
-2.46254349664406));
#369645=CARTESIAN_POINT('Ctrl Pts',(-1.2604813845259,0.014442586313074,
-2.48211655517883));
#369646=CARTESIAN_POINT('Ctrl Pts',(-1.24788218824376,0.178373896895093,
-2.49195243381375));
#369647=CARTESIAN_POINT('Ctrl Pts',(-1.16163592241478,0.488139475969799,
-2.51053836855824));
#369648=CARTESIAN_POINT('Ctrl Pts',(-1.09037690212478,0.63146750447024,
-2.51853637931777));
#369649=CARTESIAN_POINT('Ctrl Pts',(-0.892749692734237,0.890795644436746,
-2.53658523454544));
#369650=CARTESIAN_POINT('Ctrl Pts',(-0.765588978650082,1.00218666747823,
-2.54653442976229));
#369651=CARTESIAN_POINT('Ctrl Pts',(-0.480574618493332,1.16509672348177,
-2.56623151202275));
#369652=CARTESIAN_POINT('Ctrl Pts',(-0.326711235242754,1.21724071537535,
-2.57579080769599));
#369653=CARTESIAN_POINT('Ctrl Pts',(-0.111645874219062,1.24626437544745,
-2.58783664146539));
#369654=CARTESIAN_POINT('Ctrl Pts',(-0.0557979962155551,1.25,-2.59085065106785));
#369655=CARTESIAN_POINT('Ctrl Pts',(-1.42386102908179E-13,1.25000000000001,
-2.59375000000002));
#369656=CARTESIAN_POINT('Ctrl Pts',(3.74700270810992E-15,1.25000000000001,
-2.65000000000001));
#369657=CARTESIAN_POINT('Ctrl Pts',(-0.0870368365289856,1.25000000000001,
-2.64547743331006));
#369658=CARTESIAN_POINT('Ctrl Pts',(-0.174017038472817,1.24091191735034,
-2.64068516695999));
#369659=CARTESIAN_POINT('Ctrl Pts',(-0.418189121696728,1.18908380191606,
-2.62644276987895));
#369660=CARTESIAN_POINT('Ctrl Pts',(-0.56876222727317,1.12485723352674,
-2.61669196475391));
#369661=CARTESIAN_POINT('Ctrl Pts',(-0.839880964929171,0.940508819212412,
-2.59707376946936));
#369662=CARTESIAN_POINT('Ctrl Pts',(-0.957046079674429,0.820998481605603,
-2.58740038139275));
#369663=CARTESIAN_POINT('Ctrl Pts',(-1.1338694789778,0.54944959773603,-2.57006590152985));
#369664=CARTESIAN_POINT('Ctrl Pts',(-1.19428053340036,0.401584919981543,
-2.5615950951989));
#369665=CARTESIAN_POINT('Ctrl Pts',(-1.25781923999118,0.0854872513799908,
-2.5426292350828));
#369666=CARTESIAN_POINT('Ctrl Pts',(-1.25816971613052,-0.0801631234019533,
-2.53269021259589));
#369667=CARTESIAN_POINT('Ctrl Pts',(-1.19464241373935,-0.403276661186595,
-2.51330340032881));
#369668=CARTESIAN_POINT('Ctrl Pts',(-1.130947533088,-0.557441487641628,
-2.50454251301085));
#369669=CARTESIAN_POINT('Ctrl Pts',(-0.950269536212173,-0.827680662772613,
-2.48704703364496));
#369670=CARTESIAN_POINT('Ctrl Pts',(-0.836727996672834,-0.942304107899593,
-2.4777085388336));
#369671=CARTESIAN_POINT('Ctrl Pts',(-0.567499653063559,-1.1260730553892,
-2.45820595530984));
#369672=CARTESIAN_POINT('Ctrl Pts',(-0.412979789708039,-1.19144996938435,
-2.44821556026668));
#369673=CARTESIAN_POINT('Ctrl Pts',(-0.0932791076376549,-1.25676118364574,
-2.42964408910203));
#369674=CARTESIAN_POINT('Ctrl Pts',(0.0683051291320635,-1.25836539260636,
-2.42170172315597));
#369675=CARTESIAN_POINT('Ctrl Pts',(0.384901361116856,-1.20021273172363,
-2.40350632055101));
#369676=CARTESIAN_POINT('Ctrl Pts',(0.536790394902123,-1.14039721052624,
-2.39381946920623));
#369677=CARTESIAN_POINT('Ctrl Pts',(0.812709266568332,-0.964090096418552,
-2.37419309064821));
#369678=CARTESIAN_POINT('Ctrl Pts',(0.933253212969323,-0.847951376294141,
-2.36444528185314));
#369679=CARTESIAN_POINT('Ctrl Pts',(1.11775814554646,-0.581527009011775,
-2.34686539331055));
#369680=CARTESIAN_POINT('Ctrl Pts',(1.1823479907869,-0.435457656484337,
-2.33862745938907));
#369681=CARTESIAN_POINT('Ctrl Pts',(1.25476494009658,-0.121775017149212,
-2.31980650102896));
#369682=CARTESIAN_POINT('Ctrl Pts',(1.25991513645705,0.0433113316044855,
-2.30990132010374));
#369683=CARTESIAN_POINT('Ctrl Pts',(1.20580612045286,0.369277092449537,
-2.29034337445304));
#369684=CARTESIAN_POINT('Ctrl Pts',(1.1458231285194,0.526681754001067,-2.28123826363247));
#369685=CARTESIAN_POINT('Ctrl Pts',(0.97157355437601,0.802484878243874,
-2.26390989643678));
#369686=CARTESIAN_POINT('Ctrl Pts',(0.861379553736349,0.919752348254905,
-2.25466602410253));
#369687=CARTESIAN_POINT('Ctrl Pts',(0.5978826770635,1.11017193361377,-2.23526173720077));
#369688=CARTESIAN_POINT('Ctrl Pts',(0.445639208929776,1.17955841433044,
-2.22526934012143));
#369689=CARTESIAN_POINT('Ctrl Pts',(0.190878358124393,1.23905928514506,
-2.21024655187576));
#369690=CARTESIAN_POINT('Ctrl Pts',(0.0954986701827122,1.25000000000001,
-2.20496225646436));
#369691=CARTESIAN_POINT('Ctrl Pts',(-4.12170297892093E-14,1.25000000000001,
-2.20000000000001));
#369692=CARTESIAN_POINT('Origin',(0.,0.,2.95));
#369693=CARTESIAN_POINT('',(-7.57054584116654E-15,1.25000000000001,-1.69375000000002));
#369694=CARTESIAN_POINT('',(-1.42462643333128E-13,1.25000000000001,-1.75));
#369695=CARTESIAN_POINT('',(-1.5308084989342E-16,1.25000000000001,2.95));
#369696=CARTESIAN_POINT('Ctrl Pts',(-1.45369827286856E-14,1.25000000000001,
-1.69375000000002));
#369697=CARTESIAN_POINT('Ctrl Pts',(0.155286777933764,1.25000000000001,
-1.70181893767377));
#369698=CARTESIAN_POINT('Ctrl Pts',(0.309345025886403,1.22106605206648,
-1.71069205749516));
#369699=CARTESIAN_POINT('Ctrl Pts',(0.606478691077016,1.10516013999761,
-1.72960875299971));
#369700=CARTESIAN_POINT('Ctrl Pts',(0.74559126023823,1.01650974762323,-1.7394967659037));
#369701=CARTESIAN_POINT('Ctrl Pts',(0.978202071192304,0.794170145224384,
-1.75825376626453));
#369702=CARTESIAN_POINT('Ctrl Pts',(1.07083083826407,0.664000290496938,
-1.76640998257022));
#369703=CARTESIAN_POINT('Ctrl Pts',(1.20567341556416,0.369239130681009,
-1.78409565215918));
#369704=CARTESIAN_POINT('Ctrl Pts',(1.24395338002485,0.206275750069565,
-1.79387345499587));
#369705=CARTESIAN_POINT('Ctrl Pts',(1.25458873064323,-0.120805419414252,
-1.81349832516489));
#369706=CARTESIAN_POINT('Ctrl Pts',(1.22850120747155,-0.281748656109735,
-1.82315491936662));
#369707=CARTESIAN_POINT('Ctrl Pts',(1.11686342852972,-0.583852736797541,
-1.84128116420789));
#369708=CARTESIAN_POINT('Ctrl Pts',(1.03275646151661,-0.722276572455576,
-1.84925469727795));
#369709=CARTESIAN_POINT('Ctrl Pts',(0.813102736283407,-0.963793726505868,
-1.86791375426473));
#369710=CARTESIAN_POINT('Ctrl Pts',(0.678131628412114,-1.0630916610204,
-1.87790599679178));
#369711=CARTESIAN_POINT('Ctrl Pts',(0.383002849197226,-1.20054098376891,
-1.89736481768551));
#369712=CARTESIAN_POINT('Ctrl Pts',(0.22666646407795,-1.23960859735568,
-1.90666032295606));
#369713=CARTESIAN_POINT('Ctrl Pts',(-0.0984540233871174,-1.25710918060458,
-1.92407909653966));
#369714=CARTESIAN_POINT('Ctrl Pts',(-0.26424740528379,-1.23296943282957,
-1.93299161496675));
#369715=CARTESIAN_POINT('Ctrl Pts',(-0.574822733720398,-1.12201798537666,
-1.95245812584322));
#369716=CARTESIAN_POINT('Ctrl Pts',(-0.716787539462754,-1.03709317355258,
-1.96238257789092));
#369717=CARTESIAN_POINT('Ctrl Pts',(-0.955764002205384,-0.821024658166677,
-1.98128221461099));
#369718=CARTESIAN_POINT('Ctrl Pts',(-1.05193413271564,-0.693529768620369,
-1.98963821388282));
#369719=CARTESIAN_POINT('Ctrl Pts',(-1.19489887339543,-0.402735570372728,
-2.00708586577768));
#369720=CARTESIAN_POINT('Ctrl Pts',(-1.23770575764424,-0.240926756812164,
-2.01679439459131));
#369721=CARTESIAN_POINT('Ctrl Pts',(-1.25750064517564,0.086139235517628,
-2.0364183541311));
#369722=CARTESIAN_POINT('Ctrl Pts',(-1.23577670752401,0.248178869789145,
-2.04614073218739));
#369723=CARTESIAN_POINT('Ctrl Pts',(-1.13242189057427,0.552845721494632,
-2.06442074328972));
#369724=CARTESIAN_POINT('Ctrl Pts',(-1.05259819111681,0.692859611668211,
-2.07234118194101));
#369725=CARTESIAN_POINT('Ctrl Pts',(-0.840186016140514,0.940361879897444,
-2.09080351036404));
#369726=CARTESIAN_POINT('Ctrl Pts',(-0.70768418083934,1.04372697881743,
-2.10078946065677));
#369727=CARTESIAN_POINT('Ctrl Pts',(-0.415666351516008,1.18968370559345,
-2.12034185397317));
#369728=CARTESIAN_POINT('Ctrl Pts',(-0.260028950008825,1.23309638342485,
-2.12973139091717));
#369729=CARTESIAN_POINT('Ctrl Pts',(-0.0669608855494323,1.24865638160365,
-2.14023030177141));
#369730=CARTESIAN_POINT('Ctrl Pts',(-0.0334623557046908,1.25,-2.14201124499338));
#369731=CARTESIAN_POINT('Ctrl Pts',(-2.69784194983923E-13,1.25000000000001,
-2.14375000000001));
#369732=CARTESIAN_POINT('Ctrl Pts',(-4.12170297892093E-14,1.25000000000001,
-2.20000000000001));
#369733=CARTESIAN_POINT('Ctrl Pts',(-0.0647810486097229,1.25,-2.19663387797322));
#369734=CARTESIAN_POINT('Ctrl Pts',(-0.129600986562227,1.24496494293533,
-2.19311468348496));
#369735=CARTESIAN_POINT('Ctrl Pts',(-0.353256875456652,1.20984938920675,
-2.18043971598379));
#369736=CARTESIAN_POINT('Ctrl Pts',(-0.506270063531051,1.15421186913492,
-2.17081979190245));
#369737=CARTESIAN_POINT('Ctrl Pts',(-0.786493493807059,0.985597069104727,
-2.15120051134026));
#369738=CARTESIAN_POINT('Ctrl Pts',(-0.910130720092299,0.872726159978944,
-2.1413900053375));
#369739=CARTESIAN_POINT('Ctrl Pts',(-1.10183240546497,0.61120721254002,
-2.12358332514547));
#369740=CARTESIAN_POINT('Ctrl Pts',(-1.17035845423982,0.466773829291593,
-2.1155064297575));
#369741=CARTESIAN_POINT('Ctrl Pts',(-1.250989790789,0.155395450473429,-2.09682372702841));
#369742=CARTESIAN_POINT('Ctrl Pts',(-1.2605702438239,-0.00904539410554187,
-2.08695727635368));
#369743=CARTESIAN_POINT('Ctrl Pts',(-1.21566154919393,-0.334877404994928,
-2.06740735570031));
#369744=CARTESIAN_POINT('Ctrl Pts',(-1.16060197035058,-0.492883303139761,
-2.05802014830617));
#369745=CARTESIAN_POINT('Ctrl Pts',(-0.995554734047103,-0.772435597087128,
-2.04105747351995));
#369746=CARTESIAN_POINT('Ctrl Pts',(-0.889336587800216,-0.892662821719336,
-2.03193140000143));
#369747=CARTESIAN_POINT('Ctrl Pts',(-0.632717987694954,-1.09061430116893,
-2.01265856201145));
#369748=CARTESIAN_POINT('Ctrl Pts',(-0.48325231240284,-1.16457864282161,
-2.00267316745407));
#369749=CARTESIAN_POINT('Ctrl Pts',(-0.167088712669152,-1.24935288526733,
-1.98370159763342));
#369750=CARTESIAN_POINT('Ctrl Pts',(-0.00380441567397249,-1.26046862460645,
-1.97551174197542));
#369751=CARTESIAN_POINT('Ctrl Pts',(0.316647040092291,-1.21988038313864,
-1.95764294864898));
#369752=CARTESIAN_POINT('Ctrl Pts',(0.470811021249917,-1.16905823065059,
-1.94810768863248));
#369753=CARTESIAN_POINT('Ctrl Pts',(0.756950846378177,-1.00870245239308,
-1.92842875382902));
#369754=CARTESIAN_POINT('Ctrl Pts',(0.884953056591838,-0.898513754696194,
-1.91847190295098));
#369755=CARTESIAN_POINT('Ctrl Pts',(1.08484115950618,-0.64096092588016,
-1.90035882758421));
#369756=CARTESIAN_POINT('Ctrl Pts',(1.15739523816577,-0.498148242707441,
-1.89238889456246));
#369757=CARTESIAN_POINT('Ctrl Pts',(1.24627629073527,-0.189149877313387,
-1.87384899263881));
#369758=CARTESIAN_POINT('Ctrl Pts',(1.26028859049331,-0.0254767233671498,
-1.86402860340204));
#369759=CARTESIAN_POINT('Ctrl Pts',(1.22449047099654,0.300943039848027,
-1.84444341760913));
#369760=CARTESIAN_POINT('Ctrl Pts',(1.17387017787683,0.460427435436986,
-1.83487435387379));
#369761=CARTESIAN_POINT('Ctrl Pts',(1.01682426480175,0.744109680436825,
-1.8178534191738));
#369762=CARTESIAN_POINT('Ctrl Pts',(0.914329258508945,0.866988940796929,
-1.80900027369363));
#369763=CARTESIAN_POINT('Ctrl Pts',(0.66410303533597,1.07171880692443,-1.78985624175215));
#369764=CARTESIAN_POINT('Ctrl Pts',(0.517300972152133,1.14978964816988,
-1.77988605755208));
#369765=CARTESIAN_POINT('Ctrl Pts',(0.24271468140597,1.23226703832922,-1.76314381364827));
#369766=CARTESIAN_POINT('Ctrl Pts',(0.121582743043821,1.25000000000003,
-1.75631762464827));
#369767=CARTESIAN_POINT('Ctrl Pts',(-2.84286483243079E-13,1.25000000000001,
-1.75));
#369768=CARTESIAN_POINT('Origin',(0.,0.,2.95));
#369769=CARTESIAN_POINT('',(1.1164467699383E-14,1.25000000000001,-1.24375000000002));
#369770=CARTESIAN_POINT('',(-4.8787575630376E-14,1.25000000000001,-1.30000000000001));
#369771=CARTESIAN_POINT('',(-1.5308084989342E-16,1.25000000000001,2.95));
#369772=CARTESIAN_POINT('Ctrl Pts',(2.24820162486595E-14,1.25000000000001,
-1.24375000000002));
#369773=CARTESIAN_POINT('Ctrl Pts',(0.0127281062361425,1.25000000000001,
-1.24441137180058));
#369774=CARTESIAN_POINT('Ctrl Pts',(0.0254632122145805,1.24980559517503,
-1.24507893946317));
#369775=CARTESIAN_POINT('Ctrl Pts',(0.203860559145116,1.24435109304023,
-1.25451237259179));
#369776=CARTESIAN_POINT('Ctrl Pts',(0.366837339527073,1.20639085544612,
-1.26411970164188));
#369777=CARTESIAN_POINT('Ctrl Pts',(0.665567426987489,1.07048208238334,
-1.28371943551069));
#369778=CARTESIAN_POINT('Ctrl Pts',(0.79896948154755,0.974969921241595,
-1.29351657443491));
#369779=CARTESIAN_POINT('Ctrl Pts',(1.01930482958355,0.74080719754203,-1.31199041667094));
#369780=CARTESIAN_POINT('Ctrl Pts',(1.10514936595059,0.605326011347319,
-1.3199304393192));
#369781=CARTESIAN_POINT('Ctrl Pts',(1.2244338282566,0.301926367291954,-1.33813441796252));
#369782=CARTESIAN_POINT('Ctrl Pts',(1.25376969848511,0.135817983777003,
-1.34810092097341));
#369783=CARTESIAN_POINT('Ctrl Pts',(1.2456139393707,-0.191692248813633,
-1.36775153492885));
#369784=CARTESIAN_POINT('Ctrl Pts',(1.21070154737509,-0.350022539283802,
-1.37725135235706));
#369785=CARTESIAN_POINT('Ctrl Pts',(1.0820322245629,-0.646659895859928,
-1.39504959375163));
#369786=CARTESIAN_POINT('Ctrl Pts',(0.988800838246133,-0.781820332299102,
-1.40332501125674));
#369787=CARTESIAN_POINT('Ctrl Pts',(0.754117042098744,-1.01045261579018,
-1.42237850752068));
#369788=CARTESIAN_POINT('Ctrl Pts',(0.614351745382173,-1.10103371717197,
-1.43235835841358));
#369789=CARTESIAN_POINT('Ctrl Pts',(0.313379499428504,-1.220463975613,-1.4515802428166));
#369790=CARTESIAN_POINT('Ctrl Pts',(0.155954832647281,-1.2503484056177,
-1.46063589701658));
#369791=CARTESIAN_POINT('Ctrl Pts',(-0.168475210398195,-1.24962999895112,
-1.47751532875827));
#369792=CARTESIAN_POINT('Ctrl Pts',(-0.332431325582248,-1.21631678881768,
-1.48703413471358));
#369793=CARTESIAN_POINT('Ctrl Pts',(-0.635284907096783,-1.08879328545755,
-1.50659657352751));
#369794=CARTESIAN_POINT('Ctrl Pts',(-0.771678355994766,-0.996782364114874,
-1.51644411266711));
#369795=CARTESIAN_POINT('Ctrl Pts',(-0.998373503197278,-0.768702169358859,
-1.53506594389332));
#369796=CARTESIAN_POINT('Ctrl Pts',(-1.08772771993399,-0.635999235042484,
-1.54309004589749));
#369797=CARTESIAN_POINT('Ctrl Pts',(-1.2155835215503,-0.336028052942537,
-1.56108831682348));
#369798=CARTESIAN_POINT('Ctrl Pts',(-1.24961419220872,-0.170316563301853,
-1.57103100620193));
#369799=CARTESIAN_POINT('Ctrl Pts',(-1.25036462615099,0.158188737307977,
-1.59074132423851));
#369800=CARTESIAN_POINT('Ctrl Pts',(-1.21960674659214,0.317816345497064,
-1.60031898072986));
#369801=CARTESIAN_POINT('Ctrl Pts',(-1.09900788393657,0.617077459222631,
-1.61827464755339));
#369802=CARTESIAN_POINT('Ctrl Pts',(-1.01015551600508,0.753785553840078,
-1.62637434629724));
#369803=CARTESIAN_POINT('Ctrl Pts',(-0.782614867327652,0.988623438011208,
-1.64524284175127));
#369804=CARTESIAN_POINT('Ctrl Pts',(-0.645070837698452,1.08339291048551,
-1.65523292335336));
#369805=CARTESIAN_POINT('Ctrl Pts',(-0.346804125794038,1.21143226967225,
-1.67457249710571));
#369806=CARTESIAN_POINT('Ctrl Pts',(-0.189838231421895,1.24572127088795,
-1.68375735426542));
#369807=CARTESIAN_POINT('Ctrl Pts',(-0.0204217310817705,1.24987494654477,
-1.69268510412202));
#369808=CARTESIAN_POINT('Ctrl Pts',(-0.0102084025352138,1.25000000000001,
-1.69321955584437));
#369809=CARTESIAN_POINT('Ctrl Pts',(-1.49880108324397E-14,1.25000000000001,
-1.69375000000002));
#369810=CARTESIAN_POINT('Ctrl Pts',(-2.84772205816363E-13,1.25000000000001,
-1.75));
#369811=CARTESIAN_POINT('Ctrl Pts',(-0.0412379402322696,1.25,-1.74785721376956));
#369812=CARTESIAN_POINT('Ctrl Pts',(-0.082521366394907,1.2479594563662,
-1.74565084771182));
#369813=CARTESIAN_POINT('Ctrl Pts',(-0.283340441980625,1.2279881156091,
-1.7346168422278));
#369814=CARTESIAN_POINT('Ctrl Pts',(-0.4384154967692,1.18153019181367,-1.72516516829753));
#369815=CARTESIAN_POINT('Ctrl Pts',(-0.72810549192602,1.02963893727432,
-1.70555569695967));
#369816=CARTESIAN_POINT('Ctrl Pts',(-0.858802387945824,0.923452201779286,
-1.69557888496588));
#369817=CARTESIAN_POINT('Ctrl Pts',(-1.06609644115566,0.671797047142976,
-1.6772579153588));
#369818=CARTESIAN_POINT('Ctrl Pts',(-1.14292836215908,0.530649881919136,
-1.66933899291516));
#369819=CARTESIAN_POINT('Ctrl Pts',(-1.24039206079692,0.224196266994979,
-1.65095177601971));
#369820=CARTESIAN_POINT('Ctrl Pts',(-1.25898881622381,0.0614480007142603,
-1.64118688004287));
#369821=CARTESIAN_POINT('Ctrl Pts',(-1.23267628598684,-0.265449968273263,
-1.62157300190361));
#369822=CARTESIAN_POINT('Ctrl Pts',(-1.18667248152148,-0.4263592175113,
-1.61191844694933));
#369823=CARTESIAN_POINT('Ctrl Pts',(-1.03795902411092,-0.714285349565246,
-1.5946428790261));
#369824=CARTESIAN_POINT('Ctrl Pts',(-0.939236737582259,-0.839893385026882,
-1.58610737094403));
#369825=CARTESIAN_POINT('Ctrl Pts',(-0.695700049671344,-1.05140649200394,
-1.56710744022566));
#369826=CARTESIAN_POINT('Ctrl Pts',(-0.551741958562074,-1.13359398593297,
-1.55716153356893));
#369827=CARTESIAN_POINT('Ctrl Pts',(-0.239639453135485,-1.23784354146212,
-1.53781672500601));
#369828=CARTESIAN_POINT('Ctrl Pts',(-0.0745058670337822,-1.25861645548798,
-1.52912993207958));
#369829=CARTESIAN_POINT('Ctrl Pts',(0.249472744485028,-1.23525801597555,
-1.51159475642273));
#369830=CARTESIAN_POINT('Ctrl Pts',(0.405344692418652,-1.19322182775177,
-1.50223432677714));
#369831=CARTESIAN_POINT('Ctrl Pts',(0.698374746362645,-1.04995514196101,
-1.48271003795615));
#369832=CARTESIAN_POINT('Ctrl Pts',(0.831672281641646,-0.947873274054076,
-1.47272123881013));
#369833=CARTESIAN_POINT('Ctrl Pts',(1.04638590509879,-0.702259138485739,
-1.45419596759593));
#369834=CARTESIAN_POINT('Ctrl Pts',(1.12756444492058,-0.562751786731794,
-1.44626510720392));
#369835=CARTESIAN_POINT('Ctrl Pts',(1.23355811931842,-0.258895173107009,
-1.42803371038643));
#369836=CARTESIAN_POINT('Ctrl Pts',(1.25667676143754,-0.0971922309217783,
-1.41833153385532));
#369837=CARTESIAN_POINT('Ctrl Pts',(1.23980119532603,0.229906637539728,
-1.39870560174763));
#369838=CARTESIAN_POINT('Ctrl Pts',(1.19843279992721,0.392097358863673,
-1.38897415846819));
#369839=CARTESIAN_POINT('Ctrl Pts',(1.05805073920253,0.684163885447196,
-1.37145016687318));
#369840=CARTESIAN_POINT('Ctrl Pts',(0.96301458371052,0.812508070063661,
-1.36316446352059));
#369841=CARTESIAN_POINT('Ctrl Pts',(0.726072104313078,1.03059125088679,
-1.34431007571227));
#369842=CARTESIAN_POINT('Ctrl Pts',(0.58501002378196,1.11671866359526,-1.33439645261598));
#369843=CARTESIAN_POINT('Ctrl Pts',(0.293050512555949,1.22406674226904,
-1.31600534903987));
#369844=CARTESIAN_POINT('Ctrl Pts',(0.147021398436324,1.25000000000002,
-1.30763945595676));
#369845=CARTESIAN_POINT('Ctrl Pts',(-9.75608482889356E-14,1.25000000000001,
-1.30000000000001));
#369846=CARTESIAN_POINT('Origin',(0.,0.,2.95));
#369847=CARTESIAN_POINT('',(1.19827546234567E-13,1.25000000000001,-0.793750000000035));
#369848=CARTESIAN_POINT('',(1.12041877347729E-15,1.25000000000001,-0.850000000000011));
#369849=CARTESIAN_POINT('',(-1.5308084989342E-16,1.25000000000001,2.95));
#369850=CARTESIAN_POINT('Ctrl Pts',(2.39808173319028E-13,1.25000000000001,
-0.793750000000035));
#369851=CARTESIAN_POINT('Ctrl Pts',(0.0365173478034769,1.25000000000001,
-0.795647497052625));
#369852=CARTESIAN_POINT('Ctrl Pts',(0.0730723172239904,1.24839986395991,
-0.797594953062993));
#369853=CARTESIAN_POINT('Ctrl Pts',(0.274707902745124,1.23065835222477,
-0.808604490777142));
#369854=CARTESIAN_POINT('Ctrl Pts',(0.435297972263029,1.18342022225767,
-0.818366139464036));
#369855=CARTESIAN_POINT('Ctrl Pts',(0.725008495213411,1.03101104211775,
-0.837992215225356));
#369856=CARTESIAN_POINT('Ctrl Pts',(0.852115607178022,0.928725125068446,
-0.847665472014617));
#369857=CARTESIAN_POINT('Ctrl Pts',(1.05948058715358,0.682424082896479,
-0.865829503710621));
#369858=CARTESIAN_POINT('Ctrl Pts',(1.13816663450739,0.541090959828185,
-0.873784542410338));
#369859=CARTESIAN_POINT('Ctrl Pts',(1.23966034531577,0.230901071017197,
-0.892395935738997));
#369860=CARTESIAN_POINT('Ctrl Pts',(1.25933320407108,0.0643772244945477,
-0.902387366530356));
#369861=CARTESIAN_POINT('Ctrl Pts',(1.23298251531999,-0.260340540740618,
-0.921870432444466));
#369862=CARTESIAN_POINT('Ctrl Pts',(1.18965009002461,-0.415659389709601,
-0.931189563382605));
#369863=CARTESIAN_POINT('Ctrl Pts',(1.04427124475132,-0.706671991977973,
-0.948650319518707));
#369864=CARTESIAN_POINT('Ctrl Pts',(0.9416398402894,-0.838584097320959,
-0.95747848154529));
#369865=CARTESIAN_POINT('Ctrl Pts',(0.692075161884984,-1.05376307551937,
-0.976901611974373));
#369866=CARTESIAN_POINT('Ctrl Pts',(0.5480324326052,-1.1353614754684,-0.986834243740048));
#369867=CARTESIAN_POINT('Ctrl Pts',(0.242017662625025,-1.23652649733511,
-1.00577018828021));
#369868=CARTESIAN_POINT('Ctrl Pts',(0.0836508584413915,-1.25720057094587,
-1.01418735676414));
#369869=CARTESIAN_POINT('Ctrl Pts',(-0.239812722176032,-1.23792859452494,
-1.03157317673759));
#369870=CARTESIAN_POINT('Ctrl Pts',(-0.401650028505976,-1.19525567937202,
-1.04126267730588));
#369871=CARTESIAN_POINT('Ctrl Pts',(-0.695931420421101,-1.05092513450937,
-1.06088390332734));
#369872=CARTESIAN_POINT('Ctrl Pts',(-0.826190438255108,-0.951935961435196,
-1.07062203563054));
#369873=CARTESIAN_POINT('Ctrl Pts',(-1.03998665229848,-0.711611274437244,
-1.08894095339615));
#369874=CARTESIAN_POINT('Ctrl Pts',(-1.12222627208494,-0.57321047632536,
-1.09685737142051));
#369875=CARTESIAN_POINT('Ctrl Pts',(-1.23259475698515,-0.2663527696126,
-1.11526883382328));
#369876=CARTESIAN_POINT('Ctrl Pts',(-1.25707176408953,-0.0999679092363408,
-1.12525192544585));
#369877=CARTESIAN_POINT('Ctrl Pts',(-1.2397440633541,0.226263518164349,
-1.14482581108989));
#369878=CARTESIAN_POINT('Ctrl Pts',(-1.20057573536714,0.383137006547994,
-1.15423822039291));
#369879=CARTESIAN_POINT('Ctrl Pts',(-1.06352535481532,0.676985820908605,
-1.17186914925455));
#369880=CARTESIAN_POINT('Ctrl Pts',(-0.96563652366167,0.810527613814236,
-1.18038988279567));
#369881=CARTESIAN_POINT('Ctrl Pts',(-0.723501631277279,1.03251673351281,
-1.19963125446348));
#369882=CARTESIAN_POINT('Ctrl Pts',(-0.581534058121792,1.11864293190939,
-1.20959189190736));
#369883=CARTESIAN_POINT('Ctrl Pts',(-0.289985603189499,1.22460330790096,
-1.22792000529143));
#369884=CARTESIAN_POINT('Ctrl Pts',(-0.145489013964085,1.25000000000001,
-1.23619016907615));
#369885=CARTESIAN_POINT('Ctrl Pts',(2.29677388219329E-14,1.25000000000001,
-1.24375000000002));
#369886=CARTESIAN_POINT('Ctrl Pts',(-9.74220704108586E-14,1.25000000000001,
-1.30000000000001));
#369887=CARTESIAN_POINT('Ctrl Pts',(-0.0190409872021563,1.25000000000001,
-1.2990106012822));
#369888=CARTESIAN_POINT('Ctrl Pts',(-0.0380972829579135,1.24956493390915,
-1.29800735512603));
#369889=CARTESIAN_POINT('Ctrl Pts',(-0.222731980051923,1.24111397627159,
-1.28815992611069));
#369890=CARTESIAN_POINT('Ctrl Pts',(-0.385128926343269,1.20067890393287,
-1.2785084810814));
#369891=CARTESIAN_POINT('Ctrl Pts',(-0.681556641099898,1.06033714157496,
-1.25889539232875));
#369892=CARTESIAN_POINT('Ctrl Pts',(-0.813322019598976,0.962989753698685,
-1.2491282407853));
#369893=CARTESIAN_POINT('Ctrl Pts',(-1.0302354240953,0.725591051741989,
-1.23073512860368));
#369894=CARTESIAN_POINT('Ctrl Pts',(-1.11419355189862,0.588590187634581,
-1.22281541125822));
#369895=CARTESIAN_POINT('Ctrl Pts',(-1.22882546163461,0.283372076139634,
-1.20450232456852));
#369896=CARTESIAN_POINT('Ctrl Pts',(-1.25562223077578,0.117102176125761,
-1.19452613056768));
#369897=CARTESIAN_POINT('Ctrl Pts',(-1.24266769967108,-0.209771385660699,
-1.17491371686049));
#369898=CARTESIAN_POINT('Ctrl Pts',(-1.20552571858969,-0.367354877423882,
-1.1654587073547));
#369899=CARTESIAN_POINT('Ctrl Pts',(-1.07248116616986,-0.662544656832272,
-1.14774732059019));
#369900=CARTESIAN_POINT('Ctrl Pts',(-0.976832623185124,-0.796862145498132,
-1.13935184765062));
#369901=CARTESIAN_POINT('Ctrl Pts',(-0.738262791311813,-1.02205221437746,
-1.1201996934855));
#369902=CARTESIAN_POINT('Ctrl Pts',(-0.59733404065815,-1.11032074290285,
-1.11022876493836));
#369903=CARTESIAN_POINT('Ctrl Pts',(-0.295016969221521,-1.22500492444781,
-1.0910793836603));
#369904=CARTESIAN_POINT('Ctrl Pts',(-0.137369759755668,-1.25250311107604,
-1.08221303543204));
#369905=CARTESIAN_POINT('Ctrl Pts',(0.186845868943726,-1.24701759014455,
-1.06520173155863));
#369906=CARTESIAN_POINT('Ctrl Pts',(0.350311044841314,-1.21129078502437,
-1.05563602770734));
#369907=CARTESIAN_POINT('Ctrl Pts',(0.651055283763593,-1.07940213285225,
-1.03605223908526));
#369908=CARTESIAN_POINT('Ctrl Pts',(0.785908291001378,-0.985563751667752,
-1.02622991984705));
#369909=CARTESIAN_POINT('Ctrl Pts',(1.00931044594874,-0.754322872482359,
-1.00768437698481));
#369910=CARTESIAN_POINT('Ctrl Pts',(1.0968464808068,-0.620188757326572,
-0.999711325439738));
#369911=CARTESIAN_POINT('Ctrl Pts',(1.22027633890838,-0.318434680606061,
-0.981606080836504));
#369912=CARTESIAN_POINT('Ctrl Pts',(1.25188032904612,-0.152502113655608,
-0.971650126819475));
#369913=CARTESIAN_POINT('Ctrl Pts',(1.24802188377458,0.17551837181343,-0.951968897691329));
#369914=CARTESIAN_POINT('Ctrl Pts',(1.21511140908213,0.334488951887869,
-0.942430662886862));
#369915=CARTESIAN_POINT('Ctrl Pts',(1.09034364386156,0.632402229996957,
-0.924555866200313));
#369916=CARTESIAN_POINT('Ctrl Pts',(0.999241971903155,0.768311677217683,
-0.916372785615359));
#369917=CARTESIAN_POINT('Ctrl Pts',(0.768015762081745,0.999966960031412,
-0.897408260827375));
#369918=CARTESIAN_POINT('Ctrl Pts',(0.629312446831229,1.09258559884888,
-0.887422465987086));
#369919=CARTESIAN_POINT('Ctrl Pts',(0.329671299273571,1.21617780828834,
-0.868144888955655));
#369920=CARTESIAN_POINT('Ctrl Pts',(0.172459340124662,1.24821827234065,
-0.859014702009984));
#369921=CARTESIAN_POINT('Ctrl Pts',(0.00895700522214871,1.24997593707043,
-0.85046614153187));
#369922=CARTESIAN_POINT('Ctrl Pts',(0.004477996082354,1.25000000000001,
-0.850232683501933));
#369923=CARTESIAN_POINT('Ctrl Pts',(0.,1.25000000000001,-0.850000000000011));
#369924=CARTESIAN_POINT('Origin',(0.,0.,2.95));
#369925=CARTESIAN_POINT('',(3.73401184355099E-14,1.25000000000001,-0.343750000000027));
#369926=CARTESIAN_POINT('',(1.04839535402128E-13,1.25000000000001,-0.400000000000021));
#369927=CARTESIAN_POINT('',(-1.5308084989342E-16,1.25000000000001,2.95));
#369928=CARTESIAN_POINT('Ctrl Pts',(7.48333177209133E-14,1.25000000000001,
-0.343750000000027));
#369929=CARTESIAN_POINT('Ctrl Pts',(0.0590798183387906,1.25000000000001,
-0.346819877411967));
#369930=CARTESIAN_POINT('Ctrl Pts',(0.118203739862037,1.24581209387059,
-0.350017683676478));
#369931=CARTESIAN_POINT('Ctrl Pts',(0.342396087495437,1.2137553293898,-0.362628762713977));
#369932=CARTESIAN_POINT('Ctrl Pts',(0.501422074682511,1.15715155894079,
-0.372590108513402));
#369933=CARTESIAN_POINT('Ctrl Pts',(0.782302987972495,0.988096824696519,
-0.392256750921568));
#369934=CARTESIAN_POINT('Ctrl Pts',(0.902760319636144,0.879414999889457,
-0.401776352223348));
#369935=CARTESIAN_POINT('Ctrl Pts',(1.09688175758355,0.621062980984667,
-0.41961375859139));
#369936=CARTESIAN_POINT('Ctrl Pts',(1.16819441836778,0.473494446690105,
-0.427840333198619));
#369937=CARTESIAN_POINT('Ctrl Pts',(1.25107686146537,0.156690871643344,
-0.446848547701424));
#369938=CARTESIAN_POINT('Ctrl Pts',(1.26081210456799,-0.00969444195940881,
-0.45683166651759));
#369939=CARTESIAN_POINT('Ctrl Pts',(1.21594231605393,-0.330490392139359,
-0.476079423528387));
#369940=CARTESIAN_POINT('Ctrl Pts',(1.16413593700529,-0.482231152694698,
-0.485183869161707));
#369941=CARTESIAN_POINT('Ctrl Pts',(1.00310790144222,-0.764002651354767,
-0.502090159081311));
#369942=CARTESIAN_POINT('Ctrl Pts',(0.893137586098338,-0.890100582752752,
-0.511544227164456));
#369943=CARTESIAN_POINT('Ctrl Pts',(0.632419645583964,-1.09047567866554,
-0.531102781624308));
#369944=CARTESIAN_POINT('Ctrl Pts',(0.484914215223203,-1.16359546852985,
-0.540960982313552));
#369945=CARTESIAN_POINT('Ctrl Pts',(0.174538128288854,-1.24786536409498,
-0.559616693741247));
#369946=CARTESIAN_POINT('Ctrl Pts',(0.0150798860017847,-1.25991949277691,
-0.567668841354896));
#369947=CARTESIAN_POINT('Ctrl Pts',(-0.307116863691302,-1.22297551077751,
-0.585518995029937));
#369948=CARTESIAN_POINT('Ctrl Pts',(-0.466421854092992,-1.17150569243725,
-0.595340819698395));
#369949=CARTESIAN_POINT('Ctrl Pts',(-0.751660673322387,-1.01167905245061,
-0.614957062713882));
#369950=CARTESIAN_POINT('Ctrl Pts',(-0.875749745986111,-0.906400855472546,
-0.624563265978754));
#369951=CARTESIAN_POINT('Ctrl Pts',(-1.07705624390254,-0.654543977177846,
-0.642579164796146));
#369952=CARTESIAN_POINT('Ctrl Pts',(-1.15238050450015,-0.510392064237707,
-0.650626476145764));
#369953=CARTESIAN_POINT('Ctrl Pts',(-1.24541625508687,-0.197131903492209,
-0.669422085790494));
#369954=CARTESIAN_POINT('Ctrl Pts',(-1.26054739582606,-0.0305998677198683,
-0.679414007936835));
#369955=CARTESIAN_POINT('Ctrl Pts',(-1.22570860841471,0.292458283934986,
-0.698797497036126));
#369956=CARTESIAN_POINT('Ctrl Pts',(-1.17847991536056,0.446202662816261,
-0.708022159769002));
#369957=CARTESIAN_POINT('Ctrl Pts',(-1.02517732108211,0.734455413406625,
-0.725317324804424));
#369958=CARTESIAN_POINT('Ctrl Pts',(-0.917925590338391,0.864787847910805,
-0.734496822636339));
#369959=CARTESIAN_POINT('Ctrl Pts',(-0.661276644980384,1.07328691194847,
-0.75408766494954));
#369960=CARTESIAN_POINT('Ctrl Pts',(-0.515371358678158,1.15048969731129,
-0.763985209579475));
#369961=CARTESIAN_POINT('Ctrl Pts',(-0.242149779611746,1.23234648324921,
-0.780637922857629));
#369962=CARTESIAN_POINT('Ctrl Pts',(-0.121309990693237,1.25000000000001,
-0.787446547979619));
#369963=CARTESIAN_POINT('Ctrl Pts',(2.40345937596587E-13,1.25000000000001,
-0.793750000000035));
#369964=CARTESIAN_POINT('Ctrl Pts',(6.93889390390723E-16,1.25000000000001,
-0.850000000000011));
#369965=CARTESIAN_POINT('Ctrl Pts',(-0.161070456295141,1.25000000000001,
-0.841630533582966));
#369966=CARTESIAN_POINT('Ctrl Pts',(-0.320734334238032,1.21886810249861,
-0.832400198196137));
#369967=CARTESIAN_POINT('Ctrl Pts',(-0.621354677061918,1.09683306156792,
-0.813118455741421));
#369968=CARTESIAN_POINT('Ctrl Pts',(-0.759078094490395,1.00644365084719,
-0.803250454728453));
#369969=CARTESIAN_POINT('Ctrl Pts',(-0.988649420329641,0.781144304134001,
-0.784562598317619));
#369970=CARTESIAN_POINT('Ctrl Pts',(-1.07959412169325,0.649678886643446,
-0.776480733198751));
#369971=CARTESIAN_POINT('Ctrl Pts',(-1.21051709652743,0.353039718571868,
-0.758682383114453));
#369972=CARTESIAN_POINT('Ctrl Pts',(-1.24661034872577,0.189567869179206,
-0.748874072150891));
#369973=CARTESIAN_POINT('Ctrl Pts',(-1.2528498488519,-0.137428795599859,
-0.729254272264144));
#369974=CARTESIAN_POINT('Ctrl Pts',(-1.22468102346119,-0.297804126963716,
-0.719631752382311));
#369975=CARTESIAN_POINT('Ctrl Pts',(-1.10906314316296,-0.598654633471895,
-0.701580721991817));
#369976=CARTESIAN_POINT('Ctrl Pts',(-1.02286331264974,-0.736316148380509,
-0.693560052349953));
#369977=CARTESIAN_POINT('Ctrl Pts',(-0.79971284996578,-0.974893530087458,
-0.674807492725708));
#369978=CARTESIAN_POINT('Ctrl Pts',(-0.663585751690908,-1.07219633131756,
-0.664815037173834));
#369979=CARTESIAN_POINT('Ctrl Pts',(-0.367033046470049,-1.20549191785441,
-0.645406839000789));
#369980=CARTESIAN_POINT('Ctrl Pts',(-0.210400404408204,-1.24244664919953,
-0.636159326235188));
#369981=CARTESIAN_POINT('Ctrl Pts',(0.115517861008065,-1.2557624780115,
-0.618824641526355));
#369982=CARTESIAN_POINT('Ctrl Pts',(0.281789808952139,-1.22918976875112,
-0.609733465077867));
#369983=CARTESIAN_POINT('Ctrl Pts',(0.591225776742806,-1.11342710022432,
-0.59018182048498));
#369984=CARTESIAN_POINT('Ctrl Pts',(0.731730043175942,-1.02656762164794,
-0.580275220283415));
#369985=CARTESIAN_POINT('Ctrl Pts',(0.967424821284296,-0.807253702477117,
-0.561448742785417));
#369986=CARTESIAN_POINT('Ctrl Pts',(1.06176654932889,-0.678386061936249,
-0.553203163716318));
#369987=CARTESIAN_POINT('Ctrl Pts',(1.20055853238085,-0.385541243379893,
-0.535632474602934));
#369988=CARTESIAN_POINT('Ctrl Pts',(1.24104077393615,-0.223122249194351,
-0.5258873349518));
#369989=CARTESIAN_POINT('Ctrl Pts',(1.25612202631843,0.103983811598946,
-0.506260971304199));
#369990=CARTESIAN_POINT('Ctrl Pts',(1.23214798552696,0.26547389174927,-0.496571566495178));
#369991=CARTESIAN_POINT('Ctrl Pts',(1.12453189915568,0.568829763456653,
-0.478370214192732));
#369992=CARTESIAN_POINT('Ctrl Pts',(1.04251622806055,0.70802524800795,-0.470429974801382));
#369993=CARTESIAN_POINT('Ctrl Pts',(0.826384873996718,0.95247021514956,
-0.451866111196714));
#369994=CARTESIAN_POINT('Ctrl Pts',(0.692602275545821,1.05375733649945,
-0.441875949825649));
#369995=CARTESIAN_POINT('Ctrl Pts',(0.398959608144391,1.19536072578793,
-0.422369727570711));
#369996=CARTESIAN_POINT('Ctrl Pts',(0.242948921825937,1.23654700648412,
-0.413027586093006));
#369997=CARTESIAN_POINT('Ctrl Pts',(0.0555960823497595,1.24907368203338,
-0.402916646719076));
#369998=CARTESIAN_POINT('Ctrl Pts',(0.0277840398287292,1.25000000000001,
-0.401443701058694));
#369999=CARTESIAN_POINT('Ctrl Pts',(2.0983215165415E-13,1.25000000000001,
-0.400000000000021));
#370000=CARTESIAN_POINT('Origin',(0.,0.,2.95));
#370001=CARTESIAN_POINT('',(-7.654042494671E-17,1.25000000000001,0.106249999999977));
#370002=CARTESIAN_POINT('',(1.04876898677003E-13,1.25000000000001,0.0499999999999784));
#370003=CARTESIAN_POINT('',(-1.5308084989342E-16,1.25000000000001,2.95));
#370004=CARTESIAN_POINT('Ctrl Pts',(0.,1.25000000000001,0.106249999999977));
#370005=CARTESIAN_POINT('Ctrl Pts',(0.0834088693143275,1.25000000000001,
0.101915948016348));
#370006=CARTESIAN_POINT('Ctrl Pts',(0.166785812227005,1.24165359687058,
0.0973331628833295));
#370007=CARTESIAN_POINT('Ctrl Pts',(0.411738826024968,1.1918818279468,0.0831118778546601));
#370008=CARTESIAN_POINT('Ctrl Pts',(0.566342753569499,1.12665789301637,
0.0731217040800425));
#370009=CARTESIAN_POINT('Ctrl Pts',(0.835784555992207,0.943143645940193,
0.0536156699233854));
#370010=CARTESIAN_POINT('Ctrl Pts',(0.949451415498427,0.828621999182428,
0.0442737172466055));
#370011=CARTESIAN_POINT('Ctrl Pts',(1.13037087400892,0.558593324922486,
0.0267720061922665));
#370012=CARTESIAN_POINT('Ctrl Pts',(1.19420420310689,0.404549174140306,
0.018022950448395));
#370013=CARTESIAN_POINT('Ctrl Pts',(1.2580832363353,0.0815449674168411,
-0.00135730195501261));
#370014=CARTESIAN_POINT('Ctrl Pts',(1.25791345087848,-0.0841239198618764,
-0.0112974351917356));
#370015=CARTESIAN_POINT('Ctrl Pts',(1.19470875237361,-0.400310883510322,
-0.0302686530106424));
#370016=CARTESIAN_POINT('Ctrl Pts',(1.13445349055922,-0.548243673418319,
-0.0387493776684003));
#370017=CARTESIAN_POINT('Ctrl Pts',(0.957917079583416,-0.819981873941055,
-0.0560746246799611));
#370018=CARTESIAN_POINT('Ctrl Pts',(0.840879668656194,-0.939615820839286,
-0.0657450853502759));
#370019=CARTESIAN_POINT('Ctrl Pts',(0.569944260123193,-1.12426118399076,
-0.0853626630392777));
#370020=CARTESIAN_POINT('Ctrl Pts',(0.419422598591749,-1.18865152536158,
-0.0951157082427667));
#370021=CARTESIAN_POINT('Ctrl Pts',(0.104889477891838,-1.25575118075505,
-0.113472318276034));
#370022=CARTESIAN_POINT('Ctrl Pts',(-0.0559083233995013,-1.25888277588398,
-0.121388598424323));
#370023=CARTESIAN_POINT('Ctrl Pts',(-0.377203291411351,-1.2033249302256,
-0.139750310058456));
#370024=CARTESIAN_POINT('Ctrl Pts',(-0.534076587870779,-1.14237658644158,
-0.149730135966533));
#370025=CARTESIAN_POINT('Ctrl Pts',(-0.809334411153535,-0.966008315914971,
-0.169324000135528));
#370026=CARTESIAN_POINT('Ctrl Pts',(-0.926434823137354,-0.854358209189572,
-0.178758219231586));
#370027=CARTESIAN_POINT('Ctrl Pts',(-1.11399790116324,-0.590164314846684,
-0.196430099484818));
#370028=CARTESIAN_POINT('Ctrl Pts',(-1.18161572487833,-0.439409693334734,
-0.20488541839994));
#370029=CARTESIAN_POINT('Ctrl Pts',(-1.25511391105904,-0.119472629925005,
-0.224081642204524));
#370030=CARTESIAN_POINT('Ctrl Pts',(-1.25992391885208,0.0466293087341037,
-0.234047758524071));
#370031=CARTESIAN_POINT('Ctrl Pts',(-1.20592409544673,0.365231644649184,
-0.253163898678975));
#370032=CARTESIAN_POINT('Ctrl Pts',(-1.14992525470469,0.515058082995038,
-0.261949873508223));
#370033=CARTESIAN_POINT('Ctrl Pts',(-0.981240132165863,0.791918120465329,
-0.279020810713878));
#370034=CARTESIAN_POINT('Ctrl Pts',(-0.867735079639031,0.914867029055821,
-0.288607173508361));
#370035=CARTESIAN_POINT('Ctrl Pts',(-0.601922899937307,1.10753616276619,
-0.308199253535092));
#370036=CARTESIAN_POINT('Ctrl Pts',(-0.452870998658559,1.17637648246142,
-0.318009427105334));
#370037=CARTESIAN_POINT('Ctrl Pts',(-0.198077417543586,1.23821417476648,
-0.333104020712493));
#370038=CARTESIAN_POINT('Ctrl Pts',(-0.0991193281752952,1.25000000000001,
-0.338599608627669));
#370039=CARTESIAN_POINT('Ctrl Pts',(7.48333177209133E-14,1.25000000000001,
-0.343750000000027));
#370040=CARTESIAN_POINT('Ctrl Pts',(2.09485206958959E-13,1.25000000000001,
-0.400000000000021));
#370041=CARTESIAN_POINT('Ctrl Pts',(-0.136903696688647,1.25000000000001,
-0.392886275247762));
#370042=CARTESIAN_POINT('Ctrl Pts',(-0.273058001040094,1.22751495154707,
-0.385136938610113));
#370043=CARTESIAN_POINT('Ctrl Pts',(-0.558353812348898,1.13033815795081,
-0.367397229591019));
#370044=CARTESIAN_POINT('Ctrl Pts',(-0.70174819474871,1.04736472661969,
-0.357457035975991));
#370045=CARTESIAN_POINT('Ctrl Pts',(-0.943985141713251,0.834547743205648,
-0.338485525485178));
#370046=CARTESIAN_POINT('Ctrl Pts',(-1.041978547034,0.708404271325426,-0.330004256279668));
#370047=CARTESIAN_POINT('Ctrl Pts',(-1.18905932418912,0.419658566023798,
-0.312679513961568));
#370048=CARTESIAN_POINT('Ctrl Pts',(-1.23415599260509,0.258486892859228,
-0.303009213571692));
#370049=CARTESIAN_POINT('Ctrl Pts',(-1.25861492432823,-0.0684721620563943,
-0.283391670276752));
#370050=CARTESIAN_POINT('Ctrl Pts',(-1.23912692196633,-0.231024950580754,
-0.273638502965289));
#370051=CARTESIAN_POINT('Ctrl Pts',(-1.139987597103,-0.536973656436101,
-0.255281580613964));
#370052=CARTESIAN_POINT('Ctrl Pts',(-1.0623094578172,-0.677797753505098,
-0.247365286023998));
#370053=CARTESIAN_POINT('Ctrl Pts',(-0.853562419787044,-0.928280526100581,
-0.229003988572199));
#370054=CARTESIAN_POINT('Ctrl Pts',(-0.722348260470575,-1.03367082872141,
-0.219024191775315));
#370055=CARTESIAN_POINT('Ctrl Pts',(-0.431986812182885,-1.18388425517077,
-0.199430165552024));
#370056=CARTESIAN_POINT('Ctrl Pts',(-0.276746455241951,-1.22948001514874,
-0.189995767184479));
#370057=CARTESIAN_POINT('Ctrl Pts',(0.0458301644706234,-1.25983488406571,
-0.172323548276687));
#370058=CARTESIAN_POINT('Ctrl Pts',(0.210194521093855,-1.24302612505785,
-0.163868756051661));
#370059=CARTESIAN_POINT('Ctrl Pts',(0.524021402602072,-1.14672862259996,
-0.144672907871327));
#370060=CARTESIAN_POINT('Ctrl Pts',(0.670280527211671,-1.06785153907181,
-0.134706748318649));
#370061=CARTESIAN_POINT('Ctrl Pts',(0.919211696323998,-0.861798778988717,
-0.115590322541451));
#370062=CARTESIAN_POINT('Ctrl Pts',(1.02097333773227,-0.738394566236283,
-0.10680367397432));
#370063=CARTESIAN_POINT('Ctrl Pts',(1.17641517753716,-0.453887450265798,
-0.0897332470160875));
#370064=CARTESIAN_POINT('Ctrl Pts',(1.22614869806113,-0.29411765853171,
-0.0801470595120406));
#370065=CARTESIAN_POINT('Ctrl Pts',(1.26011786530385,0.032415887063119,
-0.0605550467763477));
#370066=CARTESIAN_POINT('Ctrl Pts',(1.24521853548645,0.195920544983718,
-0.0507447673011102));
#370067=CARTESIAN_POINT('Ctrl Pts',(1.1546812098639,0.504433246136558,-0.032234005231937));
#370068=CARTESIAN_POINT('Ctrl Pts',(1.0813087608889,0.646923000665087,-0.024278761356057));
#370069=CARTESIAN_POINT('Ctrl Pts',(0.879996318837545,0.903351473327351,
-0.00612540584132411));
#370070=CARTESIAN_POINT('Ctrl Pts',(0.75146843718215,1.01277802912597,0.00383589546912666));
#370071=CARTESIAN_POINT('Ctrl Pts',(0.464629472064984,1.17151740429263,
0.0235026665593323));
#370072=CARTESIAN_POINT('Ctrl Pts',(0.310281465381834,1.22150424509551,
0.0330224294720864));
#370073=CARTESIAN_POINT('Ctrl Pts',(0.100584043353169,1.24696823739944,
0.0446825469163021));
#370074=CARTESIAN_POINT('Ctrl Pts',(0.0502665808276812,1.25000000000001,
0.0473880718425048));
#370075=CARTESIAN_POINT('Ctrl Pts',(2.099068782039E-13,1.25000000000001,
0.0499999999999786));
#370076=CARTESIAN_POINT('Origin',(0.,0.,2.95));
#370077=CARTESIAN_POINT('',(-9.75093065587137E-14,1.25000000000001,0.556249999999987));
#370078=CARTESIAN_POINT('',(-7.654042494671E-17,1.25000000000001,0.499999999999989));
#370079=CARTESIAN_POINT('',(-1.5308084989342E-16,1.25000000000001,2.95));
#370080=CARTESIAN_POINT('Ctrl Pts',(-1.95538030212106E-13,1.25000000000001,
0.556249999999987));
#370081=CARTESIAN_POINT('Ctrl Pts',(0.110095727452467,1.25000000000002,
0.550529258190659));
#370082=CARTESIAN_POINT('Ctrl Pts',(0.219897164527631,1.23545967302211,
0.544387598348574));
#370083=CARTESIAN_POINT('Ctrl Pts',(0.483988304843397,1.16397911390651,
0.528520603389435));
#370084=CARTESIAN_POINT('Ctrl Pts',(0.631540368194716,1.09098321222581,
0.518663696224431));
#370085=CARTESIAN_POINT('Ctrl Pts',(0.892410668998942,0.890829214599118,
0.49910385784027));
#370086=CARTESIAN_POINT('Ctrl Pts',(1.00248282092227,0.7648221248362,0.489639327490149));
#370087=CARTESIAN_POINT('Ctrl Pts',(1.16373402854627,0.483196003908649,
0.472741760234496));
#370088=CARTESIAN_POINT('Ctrl Pts',(1.21566272275007,0.331511123020428,
0.463640667381203));
#370089=CARTESIAN_POINT('Ctrl Pts',(1.26080142902313,0.0107803782299532,
0.444396822693775));
#370090=CARTESIAN_POINT('Ctrl Pts',(1.25121127696836,-0.155598633295204,
0.434414082002265));
#370091=CARTESIAN_POINT('Ctrl Pts',(1.16860360178229,-0.472495905952001,
0.415400245642857));
#370092=CARTESIAN_POINT('Ctrl Pts',(1.09739924970882,-0.620157362400895,
0.407167816828459));
#370093=CARTESIAN_POINT('Ctrl Pts',(0.903470949119029,-0.878682593259535,
0.38933524981329));
#370094=CARTESIAN_POINT('Ctrl Pts',(0.783111943046633,-0.987453723955263,
0.379818078483398));
#370095=CARTESIAN_POINT('Ctrl Pts',(0.507349053267152,-1.1537400470651,
0.360500428711867));
#370096=CARTESIAN_POINT('Ctrl Pts',(0.354373467382822,-1.20952473987467,
0.350878043314579));
#370097=CARTESIAN_POINT('Ctrl Pts',(0.0360168821165519,-1.25980624593843,
0.332827304714507));
#370098=CARTESIAN_POINT('Ctrl Pts',(-0.126302915894441,-1.25397726122806,
0.32480642581262));
#370099=CARTESIAN_POINT('Ctrl Pts',(-0.44448908312833,-1.17999457526421,
0.306053506996264));
#370100=CARTESIAN_POINT('Ctrl Pts',(-0.596814831391358,-1.11074875148646,
0.296061054224156));
#370101=CARTESIAN_POINT('Ctrl Pts',(-0.860517304112876,-0.920561641676312,
0.276653058504795));
#370102=CARTESIAN_POINT('Ctrl Pts',(-0.970830823621374,-0.803386125286054,
0.267405734396574));
#370103=CARTESIAN_POINT('Ctrl Pts',(-1.14530928127823,-0.527779774932947,
0.250071377281343));
#370104=CARTESIAN_POINT('Ctrl Pts',(-1.20542533674739,-0.370491333408049,
0.24097948000446));
#370105=CARTESIAN_POINT('Ctrl Pts',(-1.25987147061771,-0.0446251390695866,
0.221427508344152));
#370106=CARTESIAN_POINT('Ctrl Pts',(-1.25489176136244,0.120483642117867,
0.211520981472905));
#370107=CARTESIAN_POINT('Ctrl Pts',(-1.18279045668018,0.434253498461013,
0.192694790092316));
#370108=CARTESIAN_POINT('Ctrl Pts',(-1.1183504744051,0.580386185888755,
0.184449609693465));
#370109=CARTESIAN_POINT('Ctrl Pts',(-0.934120381403464,0.846995847917418,
0.166878443391746));
#370110=CARTESIAN_POINT('Ctrl Pts',(-0.813695985431435,0.963257286950447,
0.157133165051925));
#370111=CARTESIAN_POINT('Ctrl Pts',(-0.537945249268492,1.13985516804468,
0.137506800061336));
#370112=CARTESIAN_POINT('Ctrl Pts',(-0.386101249454913,1.19982940090801,
0.127817527400389));
#370113=CARTESIAN_POINT('Ctrl Pts',(-0.15197324095669,1.24307314195488,
0.114354566983167));
#370114=CARTESIAN_POINT('Ctrl Pts',(-0.0759842892410821,1.25000000000001,
0.110198259486254));
#370115=CARTESIAN_POINT('Ctrl Pts',(0.,1.25000000000001,0.106249999999977));
#370116=CARTESIAN_POINT('Ctrl Pts',(2.11150541495897E-13,1.25000000000001,
0.0499999999999785));
#370117=CARTESIAN_POINT('Ctrl Pts',(-0.111470455421133,1.25000000000001,
0.0557921747699455));
#370118=CARTESIAN_POINT('Ctrl Pts',(-0.222643888038024,1.23509422747958,
0.0620160889577699));
#370119=CARTESIAN_POINT('Ctrl Pts',(-0.489772689440863,1.16183835855839,
0.078094184711249));
#370120=CARTESIAN_POINT('Ctrl Pts',(-0.638739409342658,1.08708482841797,
0.0880773284406671));
#370121=CARTESIAN_POINT('Ctrl Pts',(-0.894134663808368,0.88784181787852,
0.107325345459251));
#370122=CARTESIAN_POINT('Ctrl Pts',(-0.99965011951641,0.767110993144499,
0.116430014109376));
#370123=CARTESIAN_POINT('Ctrl Pts',(-1.16317318624406,0.486778909701346,
0.133336884406127));
#370124=CARTESIAN_POINT('Ctrl Pts',(-1.21740066739827,0.328495708506877,
0.14279025748945));
#370125=CARTESIAN_POINT('Ctrl Pts',(-1.26058944048159,0.00252123275269689,
0.162348726034704));
#370126=CARTESIAN_POINT('Ctrl Pts',(-1.25016901739024,-0.161783543797773,
0.172207012627734));
#370127=CARTESIAN_POINT('Ctrl Pts',(-1.16797700891844,-0.472716691392178,
0.190863001483401));
#370128=CARTESIAN_POINT('Ctrl Pts',(-1.09869491440265,-0.616841832868966,
0.198915392573041));
#370129=CARTESIAN_POINT('Ctrl Pts',(-0.90561638891264,-0.877410288353267,
0.216765100717548));
#370130=CARTESIAN_POINT('Ctrl Pts',(-0.781395758288791,-0.98964417282974,
0.226586810559507));
#370131=CARTESIAN_POINT('Ctrl Pts',(-0.500370692919775,-1.15677037951647,
0.246203087502697));
#370132=CARTESIAN_POINT('Ctrl Pts',(-0.347154646230893,-1.21160391429263,
0.255809432867983));
#370133=CARTESIAN_POINT('Ctrl Pts',(-0.0283905049197947,-1.26002830846002,
0.273825635344463));
#370134=CARTESIAN_POINT('Ctrl Pts',(0.134109254753663,-1.25319391071158,
0.281872703968469));
#370135=CARTESIAN_POINT('Ctrl Pts',(0.451921694253178,-1.17715322848757,
0.30066794320991));
#370136=CARTESIAN_POINT('Ctrl Pts',(0.603712955450508,-1.10699912270918,
0.310659871679425));
#370137=CARTESIAN_POINT('Ctrl Pts',(0.866081876952995,-0.915311906885435,
0.330043577225222));
#370138=CARTESIAN_POINT('Ctrl Pts',(0.975620884385336,-0.797543653015307,
0.339268438629833));
#370139=CARTESIAN_POINT('Ctrl Pts',(1.148616831659,-0.520664513371695,0.356563945924589));
#370140=CARTESIAN_POINT('Ctrl Pts',(1.20786977038538,-0.362622214666592,
0.365742667119868));
#370141=CARTESIAN_POINT('Ctrl Pts',(1.26013003425235,-0.0361137966221107,
0.38533317220254));
#370142=CARTESIAN_POINT('Ctrl Pts',(1.25404666538466,0.128846617713408,
0.395230797062673));
#370143=CARTESIAN_POINT('Ctrl Pts',(1.17990149401884,0.44204997373243,0.414022998423818));
#370144=CARTESIAN_POINT('Ctrl Pts',(1.11448934346675,0.587773184588203,
0.422222630516152));
#370145=CARTESIAN_POINT('Ctrl Pts',(0.928477354831601,0.853178879245708,
0.439850267809871));
#370146=CARTESIAN_POINT('Ctrl Pts',(0.807279689485484,0.968641952923779,
0.449611775444361));
#370147=CARTESIAN_POINT('Ctrl Pts',(0.530443711573877,1.14335071217548,
0.469237857595093));
#370148=CARTESIAN_POINT('Ctrl Pts',(0.378310471213608,1.20229482442116,
0.478911256017188));
#370149=CARTESIAN_POINT('Ctrl Pts',(0.146649687795479,1.24355080550249,
0.492186382859672));
#370150=CARTESIAN_POINT('Ctrl Pts',(0.0733172695478839,1.25000000000001,
0.496190322922115));
#370151=CARTESIAN_POINT('Ctrl Pts',(0.,1.25000000000001,0.499999999999989));
#370152=CARTESIAN_POINT('Origin',(0.,0.,2.95));
#370153=CARTESIAN_POINT('',(-8.24839292940005E-14,1.25000000000001,1.00624999999999));
#370154=CARTESIAN_POINT('',(-3.00232052310016E-14,1.25000000000001,0.949999999999992));
#370155=CARTESIAN_POINT('',(-1.5308084989342E-16,1.25000000000001,2.95));
#370156=CARTESIAN_POINT('Ctrl Pts',(-1.64070146357886E-13,1.25000000000001,
1.00624999999999));
#370157=CARTESIAN_POINT('Ctrl Pts',(0.132760180009687,1.25000000000002,
0.999351578690014));
#370158=CARTESIAN_POINT('Ctrl Pts',(0.264827410352974,1.22885544962755,
0.991854827589753));
#370159=CARTESIAN_POINT('Ctrl Pts',(0.546966301958247,1.13587327957377,
0.974404995636595));
#370160=CARTESIAN_POINT('Ctrl Pts',(0.691072290179626,1.05441864922568,
0.964473389927922));
#370161=CARTESIAN_POINT('Ctrl Pts',(0.940870633762533,0.839457016764246,
0.945044638272116));
#370162=CARTESIAN_POINT('Ctrl Pts',(1.04365286579185,0.707596550603973,
0.936205793036214));
#370163=CARTESIAN_POINT('Ctrl Pts',(1.18929328356091,0.416674090237899,
0.91875044541425));
#370164=CARTESIAN_POINT('Ctrl Pts',(1.23275537538807,0.261405752446612,
0.909434345146773));
#370165=CARTESIAN_POINT('Ctrl Pts',(1.25938782921475,-0.0632606126396011,
0.8899543632416));
#370166=CARTESIAN_POINT('Ctrl Pts',(1.23986538365966,-0.229786650150815,
0.879962800990927));
#370167=CARTESIAN_POINT('Ctrl Pts',(1.1386506424248,-0.540079495994821,
0.861345230240287));
#370168=CARTESIAN_POINT('Ctrl Pts',(1.06007585639613,-0.681505171105023,
0.85338800216148));
#370169=CARTESIAN_POINT('Ctrl Pts',(0.852911782822347,-0.927991634854894,
0.835228847221003));
#370170=CARTESIAN_POINT('Ctrl Pts',(0.725904037164835,-1.030378561644,0.825557723364322));
#370171=CARTESIAN_POINT('Ctrl Pts',(0.436339301598169,-1.18303677761975,
0.805931751862598));
#370172=CARTESIAN_POINT('Ctrl Pts',(0.275790164279255,-1.23041635082661,
0.796167986777961));
#370173=CARTESIAN_POINT('Ctrl Pts',(-0.047042049554638,-1.25910770535608,
0.77853239224167));
#370174=CARTESIAN_POINT('Ctrl Pts',(-0.205966929131309,-1.2430424311163,
0.770338917355434));
#370175=CARTESIAN_POINT('Ctrl Pts',(-0.514356173324183,-1.15094190380244,
0.751551526352524));
#370176=CARTESIAN_POINT('Ctrl Pts',(-0.660316890432176,-1.07387545713724,
0.741655191614361));
#370177=CARTESIAN_POINT('Ctrl Pts',(-0.917183631103573,-0.865584795699296,
0.722059284402699));
#370178=CARTESIAN_POINT('Ctrl Pts',(-1.02457899863437,-0.735301446329246,
0.712868086779731));
#370179=CARTESIAN_POINT('Ctrl Pts',(-1.17812502949243,-0.447134449431192,
0.695578066965848));
#370180=CARTESIAN_POINT('Ctrl Pts',(-1.22547236411816,-0.293439875093998,
0.686356392505617));
#370181=CARTESIAN_POINT('Ctrl Pts',(-1.260570321567,0.0295639601923402,
0.666976162388436));
#370182=CARTESIAN_POINT('Ctrl Pts',(-1.24557820086212,0.196094352339869,
0.656984338859585));
#370183=CARTESIAN_POINT('Ctrl Pts',(-1.15280253655963,0.509447233287784,
0.63818316600271));
#370184=CARTESIAN_POINT('Ctrl Pts',(-1.07758131698412,0.653686233007904,
0.630132180718844));
#370185=CARTESIAN_POINT('Ctrl Pts',(-0.876460055967045,0.905711828286041,
0.612120845583583));
#370186=CARTESIAN_POINT('Ctrl Pts',(-0.752463932383305,1.01107975625542,
0.602516780164843));
#370187=CARTESIAN_POINT('Ctrl Pts',(-0.467364233531721,1.17113014174595,
0.582901053691121));
#370188=CARTESIAN_POINT('Ctrl Pts',(-0.30810016347818,1.22272822250969,
0.573077507433621));
#370189=CARTESIAN_POINT('Ctrl Pts',(-0.0957032265067624,1.24725522245179,
0.561305228849163));
#370190=CARTESIAN_POINT('Ctrl Pts',(-0.0478281484139007,1.25,0.558735223492522));
#370191=CARTESIAN_POINT('Ctrl Pts',(-1.94865532267534E-13,1.25000000000001,
0.556249999999987));
#370192=CARTESIAN_POINT('Ctrl Pts',(0.,1.25000000000001,0.499999999999989));
#370193=CARTESIAN_POINT('Ctrl Pts',(-0.0862682746159715,1.25000000000001,
0.504482631041474));
#370194=CARTESIAN_POINT('Ctrl Pts',(-0.172487434489133,1.24107165734585,
0.50923056028556));
#370195=CARTESIAN_POINT('Ctrl Pts',(-0.419792968061261,1.18905309932987,
0.523641489500238));
#370196=CARTESIAN_POINT('Ctrl Pts',(-0.57384815019037,1.12283710963577,
0.53363291126957));
#370197=CARTESIAN_POINT('Ctrl Pts',(-0.841898962499962,0.937672385738494,
0.553116181764401));
#370198=CARTESIAN_POINT('Ctrl Pts',(-0.954750036912509,0.822491771888897,
0.562435514017028));
#370199=CARTESIAN_POINT('Ctrl Pts',(-1.13409880660983,0.551095765076556,
0.579896629663123));
#370200=CARTESIAN_POINT('Ctrl Pts',(-1.19703032424223,0.396265274860239,
0.588724083508252));
#370201=CARTESIAN_POINT('Ctrl Pts',(-1.25861872515985,0.0725526675554756,
0.608146839946541));
#370202=CARTESIAN_POINT('Ctrl Pts',(-1.25727402968328,-0.0929923270629792,
0.61807953962365));
#370203=CARTESIAN_POINT('Ctrl Pts',(-1.19189731845674,-0.408596573876534,
0.637015794432467));
#370204=CARTESIAN_POINT('Ctrl Pts',(-1.13062717708045,-0.556087186048838,
0.645433504127685));
#370205=CARTESIAN_POINT('Ctrl Pts',(-0.952221908809357,-0.826589841779339,
0.662818793469107));
#370206=CARTESIAN_POINT('Ctrl Pts',(-0.834354752304146,-0.945415787489115,
0.672508128948723));
#370207=CARTESIAN_POINT('Ctrl Pts',(-0.56223060675814,-1.12812288180903,
0.692129327159882));
#370208=CARTESIAN_POINT('Ctrl Pts',(-0.411376867902615,-1.19144538062551,
0.701867592330662));
#370209=CARTESIAN_POINT('Ctrl Pts',(-0.0963557838829768,-1.25645451633575,
0.720186842091296));
#370210=CARTESIAN_POINT('Ctrl Pts',(0.064621031364767,-1.25848548666364,
0.728103242686795));
#370211=CARTESIAN_POINT('Ctrl Pts',(0.385555073851676,-1.20065867985365,
0.746514268915072));
#370212=CARTESIAN_POINT('Ctrl Pts',(0.541891884231855,-1.13867314532483,
0.75649733391109));
#370213=CARTESIAN_POINT('Ctrl Pts',(0.815765074426867,-0.960566583942252,
0.776071399160033));
#370214=CARTESIAN_POINT('Ctrl Pts',(0.932044640374465,-0.848215269769055,
0.78548400206833));
#370215=CARTESIAN_POINT('Ctrl Pts',(1.11801415160888,-0.582614236382718,
0.803115292333425));
#370216=CARTESIAN_POINT('Ctrl Pts',(1.18472836351054,-0.431076105084149,
0.81163543369482));
#370217=CARTESIAN_POINT('Ctrl Pts',(1.25592957878956,-0.110393178259806,
0.830876409304284));
#370218=CARTESIAN_POINT('Ctrl Pts',(1.25954389228496,0.0556182878332724,
0.84083709726987));
#370219=CARTESIAN_POINT('Ctrl Pts',(1.20333352798253,0.37364868035265,0.859918920821036));
#370220=CARTESIAN_POINT('Ctrl Pts',(1.14631880003878,0.523017439510358,
0.868626051085022));
#370221=CARTESIAN_POINT('Ctrl Pts',(0.975758416920615,0.798664048580137,
0.88575802683669));
#370222=CARTESIAN_POINT('Ctrl Pts',(0.861403046258177,0.920832937256386,
0.89536517286015));
#370223=CARTESIAN_POINT('Ctrl Pts',(0.594348557227779,1.11160334448386,
0.914964843378677));
#370224=CARTESIAN_POINT('Ctrl Pts',(0.444934762586208,1.17938625870543,
0.924762099315452));
#370225=CARTESIAN_POINT('Ctrl Pts',(0.19254863413642,1.23886551112042,0.939660844815923));
#370226=CARTESIAN_POINT('Ctrl Pts',(0.0963410370308149,1.25000000000001,
0.944993972870252));
#370227=CARTESIAN_POINT('Ctrl Pts',(-5.98933296121097E-14,1.25000000000001,
0.949999999999993));
#370228=CARTESIAN_POINT('Origin',(0.,0.,2.95));
#370229=CARTESIAN_POINT('',(9.03658428620226E-9,1.25000000000001,1.45624999906087));
#370230=CARTESIAN_POINT('',(-1.20004646332587E-13,1.25000000000001,1.4));
#370231=CARTESIAN_POINT('',(-1.5308084989342E-16,1.25000000000001,2.95));
#370232=CARTESIAN_POINT('Ctrl Pts',(1.80731740684337E-8,1.25000000000001,
1.45624999906087));
#370233=CARTESIAN_POINT('Ctrl Pts',(0.157398679770193,1.24999999772425,
1.44807132461952));
#370234=CARTESIAN_POINT('Ctrl Pts',(0.313475064425583,1.22026998729107,
1.43906945746397));
#370235=CARTESIAN_POINT('Ctrl Pts',(0.613327249792887,1.10160244908175,
1.41992865472319));
#370236=CARTESIAN_POINT('Ctrl Pts',(0.753163918005052,1.01116072139918,
1.40994927646958));
#370237=CARTESIAN_POINT('Ctrl Pts',(0.988083053645535,0.782735539991384,
1.39088976466936));
#370238=CARTESIAN_POINT('Ctrl Pts',(1.08146010550208,0.64762610461839,1.38260756627708));
#370239=CARTESIAN_POINT('Ctrl Pts',(1.21039467654472,0.351076002414244,
1.36481456014483));
#370240=CARTESIAN_POINT('Ctrl Pts',(1.24544270847957,0.192790124873009,
1.35531740749235));
#370241=CARTESIAN_POINT('Ctrl Pts',(1.2538900214955,-0.134683444613013,
1.33566899332319));
#370242=CARTESIAN_POINT('Ctrl Pts',(1.22470822614229,-0.300802691914751,
1.32570183848509));
#370243=CARTESIAN_POINT('Ctrl Pts',(1.10570570688357,-0.604313394287262,
1.30749119634274));
#370244=CARTESIAN_POINT('Ctrl Pts',(1.01997583690477,-0.739886435954298,
1.29955290608169));
#370245=CARTESIAN_POINT('Ctrl Pts',(0.799848460765771,-0.974246553231572,
1.28108394857509));
#370246=CARTESIAN_POINT('Ctrl Pts',(0.666545352774837,-1.06987122986475,
1.27128857560068));
#370247=CARTESIAN_POINT('Ctrl Pts',(0.367953555362538,-1.20605101944918,
1.2516878969979));
#370248=CARTESIAN_POINT('Ctrl Pts',(0.205010971191739,-1.2441621947968,
1.24207781670246));
#370249=CARTESIAN_POINT('Ctrl Pts',(-0.118969573749707,-1.25436750783854,
1.22493713437614));
#370250=CARTESIAN_POINT('Ctrl Pts',(-0.276850276553407,-1.22921762208352,
1.21624096631008));
#370251=CARTESIAN_POINT('Ctrl Pts',(-0.580464475410518,-1.11919602198872,
1.19716406175764));
#370252=CARTESIAN_POINT('Ctrl Pts',(-0.72250095688813,-1.03321468577995,
1.18720418959795));
#370253=CARTESIAN_POINT('Ctrl Pts',(-0.964875735814266,-0.811442469879943,
1.16795686017375));
#370254=CARTESIAN_POINT('Ctrl Pts',(-1.06291611579921,-0.677952986670806,
1.15942717920022));
#370255=CARTESIAN_POINT('Ctrl Pts',(-1.20023579293853,-0.384194857888461,
1.14180169147328));
#370256=CARTESIAN_POINT('Ctrl Pts',(-1.23953981270102,-0.227369990182164,
1.1323921994109));
#370257=CARTESIAN_POINT('Ctrl Pts',(-1.25716076480177,0.0988162526587568,
1.11282102484045));
#370258=CARTESIAN_POINT('Ctrl Pts',(-1.23283951488155,0.265207716207856,
1.1028375370275));
#370259=CARTESIAN_POINT('Ctrl Pts',(-1.12275777229388,0.572174767427489,
1.08441951395433));
#370260=CARTESIAN_POINT('Ctrl Pts',(-1.04063341076924,0.710669974097316,
1.07650279896224));
#370261=CARTESIAN_POINT('Ctrl Pts',(-0.827046213520172,0.951190122724477,
1.05818887817897));
#370262=CARTESIAN_POINT('Ctrl Pts',(-0.696888708734302,1.05028835281727,
1.04845274893792));
#370263=CARTESIAN_POINT('Ctrl Pts',(-0.402752868975319,1.19488464689099,
1.02883111355203));
#370264=CARTESIAN_POINT('Ctrl Pts',(-0.240954146332926,1.23770703193248,
1.01913913375429));
#370265=CARTESIAN_POINT('Ctrl Pts',(-0.0503287006321313,1.24924080334692,
1.00888793189678));
#370266=CARTESIAN_POINT('Ctrl Pts',(-0.0251530851071151,1.25,1.00755699264116));
#370267=CARTESIAN_POINT('Ctrl Pts',(-1.64814777738108E-13,1.25000000000001,
1.00624999999999));
#370268=CARTESIAN_POINT('Ctrl Pts',(-5.98933296121097E-14,1.25000000000001,
0.949999999999993));
#370269=CARTESIAN_POINT('Ctrl Pts',(-0.0619569747754295,1.25,0.953219378845819));
#370270=CARTESIAN_POINT('Ctrl Pts',(-0.123954635380717,1.24539432313515,
0.956579042095208));
#370271=CARTESIAN_POINT('Ctrl Pts',(-0.350667273950477,1.21137547504059,
0.969379941799671));
#370272=CARTESIAN_POINT('Ctrl Pts',(-0.509193775382237,1.15373611528708,
0.979346401237057));
#370273=CARTESIAN_POINT('Ctrl Pts',(-0.788759858261056,0.982933458839484,
0.998997160719062));
#370274=CARTESIAN_POINT('Ctrl Pts',(-0.908428770459634,0.873539624078199,
1.00849715484233));
#370275=CARTESIAN_POINT('Ctrl Pts',(-1.10100341662785,0.613802400120149,
1.02629574370347));
#370276=CARTESIAN_POINT('Ctrl Pts',(-1.17144786116564,0.465488112493403,
1.03457071325027));
#370277=CARTESIAN_POINT('Ctrl Pts',(-1.25212704344905,0.147936500855631,
1.05362380994854));
#370278=CARTESIAN_POINT('Ctrl Pts',(-1.26070031217406,-0.018394865215165,
1.06360369191278));
#370279=CARTESIAN_POINT('Ctrl Pts',(-1.21366305072875,-0.338764412054756,
1.08282586472316));
#370280=CARTESIAN_POINT('Ctrl Pts',(-1.1608401142715,-0.490044425954557,
1.09188231105704));
#370281=CARTESIAN_POINT('Ctrl Pts',(-0.998019036056536,-0.770660115022403,
1.10876121312942));
#370282=CARTESIAN_POINT('Ctrl Pts',(-0.887198313757397,-0.896000136205884,
1.11827982741153));
#370283=CARTESIAN_POINT('Ctrl Pts',(-0.625343945649038,-1.09453322689978,
1.13784217222478));
#370284=CARTESIAN_POINT('Ctrl Pts',(-0.477466739633206,-1.1666569241532,
1.1476898081654));
#370285=CARTESIAN_POINT('Ctrl Pts',(-0.166600317335141,-1.2489582898092,
1.16631194226871));
#370286=CARTESIAN_POINT('Ctrl Pts',(-0.00700038512510649,-1.25999897012053,
1.17433628021498));
#370287=CARTESIAN_POINT('Ctrl Pts',(0.316712794779445,-1.22075857074284,
1.19233412243654));
#370288=CARTESIAN_POINT('Ctrl Pts',(0.477242499509596,-1.16738309297785,
1.20227675491099));
#370289=CARTESIAN_POINT('Ctrl Pts',(0.762122401229375,-1.00379534756186,
1.22198718118849));
#370290=CARTESIAN_POINT('Ctrl Pts',(0.884991537089302,-0.897350601019584,
1.23156499116451));
#370291=CARTESIAN_POINT('Ctrl Pts',(1.08387274485231,-0.643290066836535,
1.24952097788549));
#370292=CARTESIAN_POINT('Ctrl Pts',(1.15784644294826,-0.497993728927597,
1.25762037626422));
#370293=CARTESIAN_POINT('Ctrl Pts',(1.24746989975567,-0.183525205164368,
1.27648848769002));
#370294=CARTESIAN_POINT('Ctrl Pts',(1.26078035155956,-0.0170236310731421,
1.28647858213549));
#370295=CARTESIAN_POINT('Ctrl Pts',(1.22255037515762,0.305306571018055,
1.30581839426096));
#370296=CARTESIAN_POINT('Ctrl Pts',(1.17377081609769,0.458391081837177,
1.31500346491011));
#370297=CARTESIAN_POINT('Ctrl Pts',(1.01827339415832,0.743683533882543,
1.33212101203284));
#370298=CARTESIAN_POINT('Ctrl Pts',(0.910830807860765,0.871991864572587,
1.34133159884764));
#370299=CARTESIAN_POINT('Ctrl Pts',(0.653915268472853,1.07777105236075,
1.3608546975055));
#370300=CARTESIAN_POINT('Ctrl Pts',(0.507588766855547,1.15392907768717,
1.37074278632415));
#370301=CARTESIAN_POINT('Ctrl Pts',(0.236607028428954,1.23315076943472,
1.38720006124292));
#370302=CARTESIAN_POINT('Ctrl Pts',(0.118514754763226,1.25000000000003,
1.3938417926991));
#370303=CARTESIAN_POINT('Ctrl Pts',(-2.40987785282698E-13,1.25000000000001,
1.4));
#370304=CARTESIAN_POINT('Origin',(0.,0.,2.95));
#370305=CARTESIAN_POINT('',(6.739087296494E-14,1.25000000000001,1.90624999999997));
#370306=CARTESIAN_POINT('',(-2.25372062308248E-14,1.25000000000001,1.84999999999999));
#370307=CARTESIAN_POINT('',(-1.5308084989342E-16,1.25000000000001,2.95));
#370308=CARTESIAN_POINT('Ctrl Pts',(1.34934826779773E-13,1.25000000000001,
1.90624999999997));
#370309=CARTESIAN_POINT('Ctrl Pts',(0.0220641490125112,1.25000000000001,
1.90510351318651));
#370310=CARTESIAN_POINT('Ctrl Pts',(0.0441478634863414,1.2494158173731,
1.90393848424304));
#370311=CARTESIAN_POINT('Ctrl Pts',(0.225701489980945,1.23978309581366,
1.89421569943465));
#370312=CARTESIAN_POINT('Ctrl Pts',(0.382056259725138,1.20084092933029,
1.88492300228407));
#370313=CARTESIAN_POINT('Ctrl Pts',(0.67727119970412,1.06363791754484,1.86546709367459));
#370314=CARTESIAN_POINT('Ctrl Pts',(0.812311756712525,0.964458122179201,
1.855474786639));
#370315=CARTESIAN_POINT('Ctrl Pts',(1.03217352987493,0.723114940154323,
1.83681013832547));
#370316=CARTESIAN_POINT('Ctrl Pts',(1.11640454143149,0.584736554500829,
1.82883419327002));
#370317=CARTESIAN_POINT('Ctrl Pts',(1.22827946254893,0.282706754242194,
1.8107124052545));
#370318=CARTESIAN_POINT('Ctrl Pts',(1.25449128915545,0.121796612551182,
1.80105779675304));
#370319=CARTESIAN_POINT('Ctrl Pts',(1.24411798257265,-0.205281189536293,
1.78143312862779));
#370320=CARTESIAN_POINT('Ctrl Pts',(1.20596811453433,-0.368275711837578,
1.77165345728971));
#370321=CARTESIAN_POINT('Ctrl Pts',(1.0713587670456,-0.663149287941581,
1.75396104272347));
#370322=CARTESIAN_POINT('Ctrl Pts',(0.978830643778726,-0.793396141507814,
1.74580964796564));
#370323=CARTESIAN_POINT('Ctrl Pts',(0.746401283578218,-1.01591304971401,
1.72705675688831));
#370324=CARTESIAN_POINT('Ctrl Pts',(0.607371161633192,-1.1046679867251,
1.71716989172824));
#370325=CARTESIAN_POINT('Ctrl Pts',(0.300822031326495,-1.22453593311983,
1.69764509327518));
#370326=CARTESIAN_POINT('Ctrl Pts',(0.136009461171029,-1.25357347005352,
1.68842446301332));
#370327=CARTESIAN_POINT('Ctrl Pts',(-0.188800153321568,-1.24587736713163,
1.67131597727303));
#370328=CARTESIAN_POINT('Ctrl Pts',(-0.345781658244665,-1.21172279151361,
1.66213434173322));
#370329=CARTESIAN_POINT('Ctrl Pts',(-0.644132371049383,-1.08394895107769,
1.64279836872858));
#370330=CARTESIAN_POINT('Ctrl Pts',(-0.781746628810574,-0.98930770402191,
1.63280848472826));
#370331=CARTESIAN_POINT('Ctrl Pts',(-1.00950805411895,-0.754659338831184,
1.61393420295339));
#370332=CARTESIAN_POINT('Ctrl Pts',(-1.09849457327402,-0.617999115840741,
1.60582994695041));
#370333=CARTESIAN_POINT('Ctrl Pts',(-1.21934347855459,-0.318818391258399,
1.58787910347547));
#370334=CARTESIAN_POINT('Ctrl Pts',(-1.25023084516112,-0.159229393009295,
1.57830376358053));
#370335=CARTESIAN_POINT('Ctrl Pts',(-1.24975730886918,0.169248596871773,
1.55859508418767));
#370336=CARTESIAN_POINT('Ctrl Pts',(-1.21587226015212,0.33497431489362,
1.54865154110635));
#370337=CARTESIAN_POINT('Ctrl Pts',(-1.08828181784335,0.635053139877062,
1.53064681160735));
#370338=CARTESIAN_POINT('Ctrl Pts',(-0.999036985526338,0.767841680002532,
1.52262623412706));
#370339=CARTESIAN_POINT('Ctrl Pts',(-0.772539813423395,0.996112588657923,
1.50400896857181));
#370340=CARTESIAN_POINT('Ctrl Pts',(-0.636238448456786,1.08823425591884,
1.49416289187609));
#370341=CARTESIAN_POINT('Ctrl Pts',(-0.333510092793093,1.21602159134482,
1.47459904502627));
#370342=CARTESIAN_POINT('Ctrl Pts',(-0.169582503259977,1.24948034391829,
1.46507735503405));
#370343=CARTESIAN_POINT('Ctrl Pts',(-0.00258301669098132,1.24999799854518,
1.45638427752798));
#370344=CARTESIAN_POINT('Ctrl Pts',(-0.0012914578997066,1.25000000001868,
1.45631710612148));
#370345=CARTESIAN_POINT('Ctrl Pts',(1.80731730328256E-8,1.25000000000001,
1.45624999906087));
#370346=CARTESIAN_POINT('Ctrl Pts',(-2.39856211815281E-13,1.25000000000001,
1.4));
#370347=CARTESIAN_POINT('Ctrl Pts',(-0.0393195961679156,1.25,1.40204310614887));
#370348=CARTESIAN_POINT('Ctrl Pts',(-0.0786799031302476,1.24814487831034,
1.40414398134325));
#370349=CARTESIAN_POINT('Ctrl Pts',(-0.28300112969979,1.22877836477191,
1.4153418191139));
#370350=CARTESIAN_POINT('Ctrl Pts',(-0.443274061016728,1.18045660176147,
1.42511949780779));
#370351=CARTESIAN_POINT('Ctrl Pts',(-0.731861214538178,1.02614144341748,
1.44474438092743));
#370352=CARTESIAN_POINT('Ctrl Pts',(-0.858204404807066,0.923083411825348,
1.45440110661728));
#370353=CARTESIAN_POINT('Ctrl Pts',(-1.06402745181118,0.675361376603991,
1.47252764691732));
#370354=CARTESIAN_POINT('Ctrl Pts',(-1.14185924872533,0.533316303320672,
1.48050102180064));
#370355=CARTESIAN_POINT('Ctrl Pts',(-1.241209262208,0.222338201800774,1.49915970789184));
#370356=CARTESIAN_POINT('Ctrl Pts',(-1.25972732850135,0.0558009014966325,
1.50915194591009));
#370357=CARTESIAN_POINT('Ctrl Pts',(-1.23121454592064,-0.268515991300665,
1.52861095947793));
#370358=CARTESIAN_POINT('Ctrl Pts',(-1.18688771354205,-0.423444179144705,
1.53790665074857));
#370359=CARTESIAN_POINT('Ctrl Pts',(-1.03949924511053,-0.713762554541242,
1.55532575327237));
#370360=CARTESIAN_POINT('Ctrl Pts',(-0.93570609504241,-0.845277099607941,
1.56423759806116));
#370361=CARTESIAN_POINT('Ctrl Pts',(-0.684345802550768,-1.05878074353627,
1.58370377130704));
#370362=CARTESIAN_POINT('Ctrl Pts',(-0.539820130271814,-1.139272204496,
1.59362828935739));
#370363=CARTESIAN_POINT('Ctrl Pts',(-0.233215705057647,-1.23821515466295,
1.61252821113129));
#370364=CARTESIAN_POINT('Ctrl Pts',(-0.0747178744562011,-1.25776237786808,
1.62088467402009));
#370365=CARTESIAN_POINT('Ctrl Pts',(0.248600826170604,-1.23619451214554,
1.63833184248745));
#370366=CARTESIAN_POINT('Ctrl Pts',(0.410137222062212,-1.19237103518111,
1.64804022414506));
#370367=CARTESIAN_POINT('Ctrl Pts',(0.703291087901194,-1.04599702234766,
1.66766416623212));
#370368=CARTESIAN_POINT('Ctrl Pts',(0.832765775709602,-0.946170315616422,
1.6773866695614));
#370369=CARTESIAN_POINT('Ctrl Pts',(1.04495034516535,-0.704340870465485,
1.69566698656232));
#370370=CARTESIAN_POINT('Ctrl Pts',(1.12630111160027,-0.565210360485072,
1.70358737837078));
#370371=CARTESIAN_POINT('Ctrl Pts',(1.23445580820926,-0.257511520102835,
1.72204930879372));
#370372=CARTESIAN_POINT('Ctrl Pts',(1.25773119996678,-0.09107935617977,
1.7320352386291));
#370373=CARTESIAN_POINT('Ctrl Pts',(1.2381423983534,0.234796739196575,1.75158780435168));
#370374=CARTESIAN_POINT('Ctrl Pts',(1.19792844216626,0.391292042360348,
1.76097752254151));
#370375=CARTESIAN_POINT('Ctrl Pts',(1.05879936094225,0.684439091728722,
1.77856634550362));
#370376=CARTESIAN_POINT('Ctrl Pts',(0.959737623783481,0.817576508230252,
1.78715786545694));
#370377=CARTESIAN_POINT('Ctrl Pts',(0.715750379695562,1.03788568616187,
1.80644508988966));
#370378=CARTESIAN_POINT('Ctrl Pts',(0.573253984920157,1.12289098212861,
1.81639957863806));
#370379=CARTESIAN_POINT('Ctrl Pts',(0.28392458895852,1.22566437795554,1.83451677693073));
#370380=CARTESIAN_POINT('Ctrl Pts',(0.142419898735792,1.25000000000001,
1.84259964498141));
#370381=CARTESIAN_POINT('Ctrl Pts',(-4.44783099240453E-14,1.25000000000001,
1.84999999999999));
#370382=CARTESIAN_POINT('Origin',(0.,0.,2.95));
#370383=CARTESIAN_POINT('',(1.34858286354831E-13,1.25000000000001,2.35624999999996));
#370384=CARTESIAN_POINT('',(-7.654042494671E-17,1.25000000000001,2.29999999999999));
#370385=CARTESIAN_POINT('',(-1.5308084989342E-16,1.25000000000001,2.95));
#370386=CARTESIAN_POINT('Ctrl Pts',(2.69869653559555E-13,1.25000000000001,
2.35624999999996));
#370387=CARTESIAN_POINT('Ctrl Pts',(0.044433163138449,1.25000000000001,
2.35394118511707));
#370388=CARTESIAN_POINT('Ctrl Pts',(0.0889145499349906,1.24763102082333,
2.35155879508408));
#370389=CARTESIAN_POINT('Ctrl Pts',(0.292891387862558,1.2257611260194,2.34030375083423));
#370390=CARTESIAN_POINT('Ctrl Pts',(0.44771822940789,1.17805333018664,2.33082747828129));
#370391=CARTESIAN_POINT('Ctrl Pts',(0.736417365076694,1.02373303828326,
2.3111966223918));
#370392=CARTESIAN_POINT('Ctrl Pts',(0.866355583473318,0.916395130127912,
2.3012246972639));
#370393=CARTESIAN_POINT('Ctrl Pts',(1.07153750812881,0.663044844477098,
2.28296262314544));
#370394=CARTESIAN_POINT('Ctrl Pts',(1.14714353414279,0.521425998584306,
2.27503555991502));
#370395=CARTESIAN_POINT('Ctrl Pts',(1.24216677553308,0.214241724025496,
2.2566045034415));
#370396=CARTESIAN_POINT('Ctrl Pts',(1.25946313075807,0.0512174419276202,
2.24682304651562));
#370397=CARTESIAN_POINT('Ctrl Pts',(1.23045164409321,-0.275572672931196,
2.2272156396241));
#370398=CARTESIAN_POINT('Ctrl Pts',(1.18312992230814,-0.436090455363154,
2.21758457267818));
#370399=CARTESIAN_POINT('Ctrl Pts',(1.0320420154748,-0.72281761118703,2.20038094332875));
#370400=CARTESIAN_POINT('Ctrl Pts',(0.932253777922101,-0.847647473052605,
2.19176190307566));
#370401=CARTESIAN_POINT('Ctrl Pts',(0.686820365306802,-1.05724974831533,
2.17272074060204));
#370402=CARTESIAN_POINT('Ctrl Pts',(0.542046066061274,-1.13828215032821,
2.16276707528395));
#370403=CARTESIAN_POINT('Ctrl Pts',(0.22932722660143,-1.23973872013907,
2.14347403063677));
#370404=CARTESIAN_POINT('Ctrl Pts',(0.0644657010172478,-1.25911568572811,
2.13487320665703));
#370405=CARTESIAN_POINT('Ctrl Pts',(-0.259026376116058,-1.23330572766472,
2.1172897665119));
#370406=CARTESIAN_POINT('Ctrl Pts',(-0.414686589460496,-1.1900238484095,
2.10790296818736));
#370407=CARTESIAN_POINT('Ctrl Pts',(-0.706801671398365,-1.04432253623698,
2.08835318391498));
#370408=CARTESIAN_POINT('Ctrl Pts',(-0.839379654808393,-0.941079165393031,
2.07836692869273));
#370409=CARTESIAN_POINT('Ctrl Pts',(-1.05201080633447,-0.69375603870744,
2.05989859616071));
#370410=CARTESIAN_POINT('Ctrl Pts',(-1.13196320875619,-0.553790353984001,
2.05197742123901));
#370411=CARTESIAN_POINT('Ctrl Pts',(-1.23556938761572,-0.249200461310902,
2.03370202767862));
#370412=CARTESIAN_POINT('Ctrl Pts',(-1.25742635352416,-0.0871923884049848,
2.02398154330427));
#370413=CARTESIAN_POINT('Ctrl Pts',(-1.23790957988289,0.239877866056647,
2.00435732803657));
#370414=CARTESIAN_POINT('Ctrl Pts',(-1.19523956098039,0.401723623453222,
1.99464658259278));
#370415=CARTESIAN_POINT('Ctrl Pts',(-1.05252064112392,0.692639357327156,
1.97719163856034));
#370416=CARTESIAN_POINT('Ctrl Pts',(-0.956458771175397,0.820215036291892,
1.96884260452183));
#370417=CARTESIAN_POINT('Ctrl Pts',(-0.717676298548484,1.03647614944333,
1.94994726989089));
#370418=CARTESIAN_POINT('Ctrl Pts',(-0.575797232204222,1.12151614880628,
1.94002381736684));
#370419=CARTESIAN_POINT('Ctrl Pts',(-0.286113450961956,1.22529191614851,
1.92185813352936));
#370420=CARTESIAN_POINT('Ctrl Pts',(-0.143508577417465,1.25000000000001,
1.91370692442225));
#370421=CARTESIAN_POINT('Ctrl Pts',(1.34441069388203E-13,1.25000000000001,
1.90624999999997));
#370422=CARTESIAN_POINT('Ctrl Pts',(-4.49213316117562E-14,1.25000000000001,
1.84999999999999));
#370423=CARTESIAN_POINT('Ctrl Pts',(-0.0157044861541279,1.25000000000001,
1.85081602903776));
#370424=CARTESIAN_POINT('Ctrl Pts',(-0.0314191927020232,1.24970404498241,
1.8516414677932));
#370425=CARTESIAN_POINT('Ctrl Pts',(-0.212761819155421,1.2428609839098,
1.86126959890323));
#370426=CARTESIAN_POINT('Ctrl Pts',(-0.375470118394336,1.20373310983395,
1.87089800635836));
#370427=CARTESIAN_POINT('Ctrl Pts',(-0.6731232162385,1.06572999251169,1.89050460853292));
#370428=CARTESIAN_POINT('Ctrl Pts',(-0.805756883777148,0.969349409244335,
1.90028787356008));
#370429=CARTESIAN_POINT('Ctrl Pts',(-1.02448095042294,0.733659818577383,
1.91872379716814));
#370430=CARTESIAN_POINT('Ctrl Pts',(-1.10943718024133,0.597465274702968,
1.92665208351771));
#370431=CARTESIAN_POINT('Ctrl Pts',(-1.22653449491264,0.293207005417949,
1.94490757967481));
#370432=CARTESIAN_POINT('Ctrl Pts',(-1.25467582129209,0.127017989629909,
1.9548789206221));
#370433=CARTESIAN_POINT('Ctrl Pts',(-1.24426086020019,-0.200201328686394,
1.97451207972108));
#370434=CARTESIAN_POINT('Ctrl Pts',(-1.20829802228421,-0.358184229595967,
1.98399105377565));
#370435=CARTESIAN_POINT('Ctrl Pts',(-1.07757143364063,-0.65414313490744,
2.00174858809434));
#370436=CARTESIAN_POINT('Ctrl Pts',(-0.983207316756803,-0.788907683287219,
2.01007827968862));
#370437=CARTESIAN_POINT('Ctrl Pts',(-0.746697357985156,-1.01592835213342,
2.02917831770666));
#370438=CARTESIAN_POINT('Ctrl Pts',(-0.60638131509394,-1.10542566430186,
2.03915427253386));
#370439=CARTESIAN_POINT('Ctrl Pts',(-0.304774524172768,-1.2226275299057,
2.05834227707547));
#370440=CARTESIAN_POINT('Ctrl Pts',(-0.147247229315901,-1.2513920043842,
2.0673070493949));
#370441=CARTESIAN_POINT('Ctrl Pts',(0.177085201866623,-1.24843996704571,
2.08424841799557));
#370442=CARTESIAN_POINT('Ctrl Pts',(0.340815911920561,-1.21399527196157,
2.09378945610528));
#370443=CARTESIAN_POINT('Ctrl Pts',(0.642689307430307,-1.08442272513257,
2.11336243426444));
#370444=CARTESIAN_POINT('Ctrl Pts',(0.778364150743864,-0.991552687290698,
2.12319840705753));
#370445=CARTESIAN_POINT('Ctrl Pts',(1.0035182001428,-0.761990269780845,
2.1417846271755));
#370446=CARTESIAN_POINT('Ctrl Pts',(1.09202120709043,-0.628619487024861,
2.1497828307784));
#370447=CARTESIAN_POINT('Ctrl Pts',(1.2178089173922,-0.327811906339744,
2.16783128561951));
#370448=CARTESIAN_POINT('Ctrl Pts',(1.25070509520255,-0.161992817094826,
2.17778043097421));
#370449=CARTESIAN_POINT('Ctrl Pts',(1.24929940706568,0.166293693894003,
2.19747762163354));
#370450=CARTESIAN_POINT('Ctrl Pts',(1.21753379203214,0.325617743326955,
2.20703706459952));
#370451=CARTESIAN_POINT('Ctrl Pts',(1.09498652619744,0.624250917867314,
2.22495505507194));
#370452=CARTESIAN_POINT('Ctrl Pts',(1.00508626477818,0.760585901245542,
2.2330917627397));
#370453=CARTESIAN_POINT('Ctrl Pts',(0.775824314847745,0.993942399079391,
2.25200525804037));
#370454=CARTESIAN_POINT('Ctrl Pts',(0.637735382131881,1.08771006731678,
2.2619935995103));
#370455=CARTESIAN_POINT('Ctrl Pts',(0.338819367231804,1.21367630871059,
2.2813047185022));
#370456=CARTESIAN_POINT('Ctrl Pts',(0.181734697085463,1.24691633605466,
2.29046427821604));
#370457=CARTESIAN_POINT('Ctrl Pts',(0.0150734947248369,1.24993186207365,
2.29921471410078));
#370458=CARTESIAN_POINT('Ctrl Pts',(0.00753536179884883,1.25000000000001,
2.29960845111532));
#370459=CARTESIAN_POINT('Ctrl Pts',(0.,1.25000000000001,2.29999999999999));
#370460=CARTESIAN_POINT('Origin',(0.,-9.76875228502569E-17,-3.6625));
#370461=CARTESIAN_POINT('',(-0.155365792422873,-0.945030276552907,-3.95478357377727));
#370462=CARTESIAN_POINT('Origin',(-4.58730275987307E-13,1.7608137170555E-12,
-3.95478357377551));
#370463=CARTESIAN_POINT('Ctrl Pts',(-0.155365792422871,-0.945030276552904,
-3.95478357377728));
#370464=CARTESIAN_POINT('Ctrl Pts',(-0.0279053867386288,-0.989345562927712,
-3.93173259563576));
#370465=CARTESIAN_POINT('Ctrl Pts',(0.0908406055947738,-0.997960828573256,
-3.91446248497396));
#370466=CARTESIAN_POINT('Ctrl Pts',(0.2939266609703,-0.994471102906672,
-3.88139632958021));
#370467=CARTESIAN_POINT('Ctrl Pts',(0.404737306683732,-0.974830092903115,
-3.86277453676972));
#370468=CARTESIAN_POINT('Ctrl Pts',(0.634402236959834,-0.895212934293821,
-3.82294769474439));
#370469=CARTESIAN_POINT('Ctrl Pts',(0.749402513368721,-0.829536503600064,
-3.80217950070126));
#370470=CARTESIAN_POINT('Ctrl Pts',(0.984142487761137,-0.630335856567594,
-3.75689034668222));
#370471=CARTESIAN_POINT('Ctrl Pts',(1.06926532203318,-0.500451973862013,
-3.73786753572628));
#370472=CARTESIAN_POINT('Ctrl Pts',(1.18794310478873,-0.270780370964604,
-3.7018818371992));
#370473=CARTESIAN_POINT('Ctrl Pts',(1.23047313162925,-0.137550427674414,
-3.68202686837076));
#370474=CARTESIAN_POINT('Ctrl Pts',(1.24999999999999,-1.42247325030098E-15,
-3.66250000000002));
#370475=CARTESIAN_POINT('',(-2.5977107395931E-13,1.07169464481439,-3.84080535518562));
#370476=CARTESIAN_POINT('Ctrl Pts',(0.875786586620195,-0.891906864368513,
-3.6624999999954));
#370477=CARTESIAN_POINT('Ctrl Pts',(0.803162978577988,-0.958147518332696,
-3.66611783025492));
#370478=CARTESIAN_POINT('Ctrl Pts',(0.7229160327686,-1.01549113836917,-3.66984833805803));
#370479=CARTESIAN_POINT('Ctrl Pts',(0.551640702174221,-1.10937740583169,
-3.67733818712611));
#370480=CARTESIAN_POINT('Ctrl Pts',(0.46136363988503,-1.14584661025103,
-3.68107032221587));
#370481=CARTESIAN_POINT('Ctrl Pts',(0.220775486284481,-1.21150525514029,
-3.69049017126946));
#370482=CARTESIAN_POINT('Ctrl Pts',(0.0667413551172497,-1.22437521577925,
-3.69573027211842));
#370483=CARTESIAN_POINT('Ctrl Pts',(-0.240687585667333,-1.19202036778278,
-3.70662761066056));
#370484=CARTESIAN_POINT('Ctrl Pts',(-0.392307468273431,-1.14470527425269,
-3.71268458241303));
#370485=CARTESIAN_POINT('Ctrl Pts',(-0.662432154086964,-0.997083129168331,
-3.72491348355897));
#370486=CARTESIAN_POINT('Ctrl Pts',(-0.779641139378463,-0.900461687408625,
-3.73095969955023));
#370487=CARTESIAN_POINT('Ctrl Pts',(-0.945919539367262,-0.699864947625556,
-3.74096526360374));
#370488=CARTESIAN_POINT('Ctrl Pts',(-1.03886893322305,-0.56454169648239,
-3.74641423599297));
#370489=CARTESIAN_POINT('Ctrl Pts',(-1.13927032774389,-0.231646122171666,
-3.75989697957764));
#370490=CARTESIAN_POINT('Ctrl Pts',(-1.15366319118036,-0.0787124006907397,
-3.76618339589642));
#370491=CARTESIAN_POINT('Ctrl Pts',(-1.12285379978883,0.212860456164627,
-3.77837702194193));
#370492=CARTESIAN_POINT('Ctrl Pts',(-1.0821482238887,0.349228633959777,
-3.78417389022775));
#370493=CARTESIAN_POINT('Ctrl Pts',(-0.950436071606793,0.60543400761943,
-3.79522025808186));
#370494=CARTESIAN_POINT('Ctrl Pts',(-0.859180942083836,0.720913828422761,
-3.80059269283917));
#370495=CARTESIAN_POINT('Ctrl Pts',(-0.64028655446859,0.905058775893708,
-3.81259207988882));
#370496=CARTESIAN_POINT('Ctrl Pts',(-0.517800650893318,0.973476873865921,
-3.81866376976776));
#370497=CARTESIAN_POINT('Ctrl Pts',(-0.24560153936023,1.06350276870297,
-3.83102133314356));
#370498=CARTESIAN_POINT('Ctrl Pts',(-0.112468620062744,1.07601604072728,
-3.83648395927268));
#370499=CARTESIAN_POINT('Ctrl Pts',(-5.19688458933132E-13,1.07169464481439,
-3.84080535518562));
#370500=CARTESIAN_POINT('',(-1.11749020422196E-16,0.912499999999999,-4.00000000000001));
#370501=CARTESIAN_POINT('',(-1.5308084989342E-16,1.25000000000001,-3.6625));
#370502=CARTESIAN_POINT('Origin',(0.,-1.02673464470213E-16,-4.00000000000001));
#370503=CARTESIAN_POINT('Ctrl Pts',(-5.19624170088432E-13,1.07169464481439,
-3.84080535518562));
#370504=CARTESIAN_POINT('Ctrl Pts',(0.0132807037919846,1.07118435866472,
-3.84131564133529));
#370505=CARTESIAN_POINT('Ctrl Pts',(0.0262725682478854,1.07043200166311,
-3.84182103819358));
#370506=CARTESIAN_POINT('Ctrl Pts',(0.164982451660776,1.05991889326409,
-3.84727828766257));
#370507=CARTESIAN_POINT('Ctrl Pts',(0.288230522434384,1.02763979747026,
-3.85269578885312));
#370508=CARTESIAN_POINT('Ctrl Pts',(0.525243537044531,0.917015259508444,
-3.864379774694));
#370509=CARTESIAN_POINT('Ctrl Pts',(0.635518934908194,0.836644670589503,
-3.87057106866854));
#370510=CARTESIAN_POINT('Ctrl Pts',(0.811012773854783,0.64746200723685,
-3.88202106240099));
#370511=CARTESIAN_POINT('Ctrl Pts',(0.889005880992891,0.531601381546978,
-3.88742893998826));
#370512=CARTESIAN_POINT('Ctrl Pts',(0.982611668862114,0.276475013801935,
-3.89912755433172));
#370513=CARTESIAN_POINT('Ctrl Pts',(1.00330564083417,0.154442537046033,
-3.90480655630969));
#370514=CARTESIAN_POINT('Ctrl Pts',(0.999305789144461,-0.0998950462085405,
-3.91685903687869));
#370515=CARTESIAN_POINT('Ctrl Pts',(0.971246564415423,-0.229819589385441,
-3.92313678730786));
#370516=CARTESIAN_POINT('Ctrl Pts',(0.886252493360822,-0.425561051651668,
-3.93276679919375));
#370517=CARTESIAN_POINT('Ctrl Pts',(0.837759723201096,-0.51280233158914,
-3.93678750846591));
#370518=CARTESIAN_POINT('Ctrl Pts',(0.70522478018958,-0.666965853173508,
-3.94601792006284));
#370519=CARTESIAN_POINT('Ctrl Pts',(0.637118232403117,-0.726582133647196,
-3.95034126928747));
#370520=CARTESIAN_POINT('Ctrl Pts',(0.561651082536775,-0.775737593869401,
-3.95478357377719));
#370521=CARTESIAN_POINT('Origin',(0.,0.,2.95));
#370522=CARTESIAN_POINT('',(1.08253175473061,0.625000000000032,2.67500000000004));
#370523=CARTESIAN_POINT('Ctrl Pts',(5.20417042793042E-16,1.25000000000001,
2.29999999999999));
#370524=CARTESIAN_POINT('Ctrl Pts',(-0.15798414204464,1.25000000000001,
2.30820909682433));
#370525=CARTESIAN_POINT('Ctrl Pts',(-0.314658277380827,1.22005106146879,
2.3172485918592));
#370526=CARTESIAN_POINT('Ctrl Pts',(-0.613432363236355,1.10130056988825,
2.33633586350722));
#370527=CARTESIAN_POINT('Ctrl Pts',(-0.751899539744469,1.01183633973303,
2.34621475595866));
#370528=CARTESIAN_POINT('Ctrl Pts',(-0.983093567839997,0.788114405040584,
2.36493960809148));
#370529=CARTESIAN_POINT('Ctrl Pts',(-1.07493687987653,0.657342186486791,
2.37305946881069));
#370530=CARTESIAN_POINT('Ctrl Pts',(-1.20795581572139,0.361704284892804,
2.39079774290633));
#370531=CARTESIAN_POINT('Ctrl Pts',(-1.24521846245067,0.198500395363415,
2.40058997627809));
#370532=CARTESIAN_POINT('Ctrl Pts',(-1.25380644971248,-0.12854883069771,
2.42021292984176));
#370533=CARTESIAN_POINT('Ctrl Pts',(-1.22674852580128,-0.289230934492819,
2.42985385606947));
#370534=CARTESIAN_POINT('Ctrl Pts',(-1.11325757004244,-0.590753157646939,
2.44794518945872));
#370535=CARTESIAN_POINT('Ctrl Pts',(-1.02817905034803,-0.728821931999858,
2.45593890732547));
#370536=CARTESIAN_POINT('Ctrl Pts',(-0.806898504343732,-0.968975574709854,
2.47464159105895));
#370537=CARTESIAN_POINT('Ctrl Pts',(-0.671386595342725,-1.06734780968674,
2.48463416345087));
#370538=CARTESIAN_POINT('Ctrl Pts',(-0.375588931227746,-1.20286831517439,
2.50406987610572));
#370539=CARTESIAN_POINT('Ctrl Pts',(-0.219111339884313,-1.24095410198731,
2.5133432638637));
#370540=CARTESIAN_POINT('Ctrl Pts',(0.106381404288763,-1.25651181033803,
2.53072309422631));
#370541=CARTESIAN_POINT('Ctrl Pts',(0.272396301628041,-1.23124542513271,
2.53971676427232));
#370542=CARTESIAN_POINT('Ctrl Pts',(0.582447754407332,-1.11806263459385,
2.55922299406372));
#370543=CARTESIAN_POINT('Ctrl Pts',(0.723738224576676,-1.03223737104514,
2.56913942015894));
#370544=CARTESIAN_POINT('Ctrl Pts',(0.961193549459415,-0.814661185400381,
2.58800524634503));
#370545=CARTESIAN_POINT('Ctrl Pts',(1.05651539179714,-0.686531607242866,
2.59630810356532));
#370546=CARTESIAN_POINT('Ctrl Pts',(1.19754974404801,-0.394785470141088,
2.61381287179143));
#370547=CARTESIAN_POINT('Ctrl Pts',(1.23928155555513,-0.232689903651711,
2.6235386057808));
#370548=CARTESIAN_POINT('Ctrl Pts',(1.25478281639912,0.0551969019069727,
2.64081181411432));
#370549=CARTESIAN_POINT('Ctrl Pts',(1.24333250688269,0.17791489555393,2.64817489373322));
#370550=CARTESIAN_POINT('Ctrl Pts',(1.18605566680237,0.412076722424357,
2.66222460334545));
#370551=CARTESIAN_POINT('Ctrl Pts',(1.14170784117889,0.522504011678397,
2.66885024070069));
#370552=CARTESIAN_POINT('Ctrl Pts',(1.08253175473058,0.624999999999965,
2.67499999999999));
#370553=CARTESIAN_POINT('',(1.21030729568997,-0.312499999999427,2.67500000000001));
#370554=CARTESIAN_POINT('Origin',(0.,1.19785708548589E-17,2.67500000000001));
#370555=CARTESIAN_POINT('Ctrl Pts',(1.21030729568997,-0.312499999999433,
2.67500000000001));
#370556=CARTESIAN_POINT('Ctrl Pts',(1.175718981605,-0.446459964424188,2.66696240213453));
#370557=CARTESIAN_POINT('Ctrl Pts',(1.11915142536756,-0.573695925916809,
2.65969193612545));
#370558=CARTESIAN_POINT('Ctrl Pts',(0.965151072782271,-0.806771638479094,
2.64469757169674));
#370559=CARTESIAN_POINT('Ctrl Pts',(0.868041694629622,-0.910432845154661,
2.63654178419092));
#370560=CARTESIAN_POINT('Ctrl Pts',(0.624071847967031,-1.09560447505936,
2.61830959019575));
#370561=CARTESIAN_POINT('Ctrl Pts',(0.473899543568118,-1.16843452864645,
2.60832150675488));
#370562=CARTESIAN_POINT('Ctrl Pts',(0.157230972575195,-1.25059130591894,
2.58940222181311));
#370563=CARTESIAN_POINT('Ctrl Pts',(-0.00581482137773669,-1.26042122838038,
2.58126048986948));
#370564=CARTESIAN_POINT('Ctrl Pts',(-0.325767666610162,-1.21749197202904,
2.56334737465988));
#370565=CARTESIAN_POINT('Ctrl Pts',(-0.479659736469491,-1.16547197089985,
2.55379030810965));
#370566=CARTESIAN_POINT('Ctrl Pts',(-0.7647806647957,-1.00280132258151,
2.53409487063524));
#370567=CARTESIAN_POINT('Ctrl Pts',(-0.892020816335206,-0.891522885192972,
2.5241449252967));
#370568=CARTESIAN_POINT('Ctrl Pts',(-1.08986046956139,-0.632361074998956,
2.5060900210567));
#370569=CARTESIAN_POINT('Ctrl Pts',(-1.16124097803301,-0.489081617941554,
2.49809489707646));
#370570=CARTESIAN_POINT('Ctrl Pts',(-1.24773512440905,-0.179387936090198,
2.47951327616538));
#370571=CARTESIAN_POINT('Ctrl Pts',(-1.26046736614005,-0.0154803948659127,
2.46967882369192));
#370572=CARTESIAN_POINT('Ctrl Pts',(-1.22203528254611,0.310757366402179,
2.45010455801583));
#370573=CARTESIAN_POINT('Ctrl Pts',(-1.170140724678,0.469821795044816,2.44056069229728));
#370574=CARTESIAN_POINT('Ctrl Pts',(-1.0107864054522,0.752310445892212,
2.42361137324643));
#370575=CARTESIAN_POINT('Ctrl Pts',(-0.907229871159249,0.874434395171338,
2.41465801507458));
#370576=CARTESIAN_POINT('Ctrl Pts',(-0.655133943368811,1.07724588582535,
2.39547438169554));
#370577=CARTESIAN_POINT('Ctrl Pts',(-0.50755464776196,1.15414494620869,
2.38549896473995));
#370578=CARTESIAN_POINT('Ctrl Pts',(-0.235584599701466,1.23330008226491,
2.36899233241693));
#370579=CARTESIAN_POINT('Ctrl Pts',(-0.117988461920189,1.25000000000001,
2.36238086032257));
#370580=CARTESIAN_POINT('Ctrl Pts',(2.69541333697276E-13,1.25000000000001,
2.35624999999996));
#370581=CARTESIAN_POINT('Origin',(0.,2.73795905253904E-16,4.));
#370582=CARTESIAN_POINT('',(-0.750000000000001,-0.433012701892221,4.));
#370583=CARTESIAN_POINT('',(-0.750000000000004,0.433012701892217,4.));
#370584=CARTESIAN_POINT('Ctrl Pts',(-0.750000000000001,-0.433012701891379,
3.99999999999958));
#370585=CARTESIAN_POINT('Ctrl Pts',(-0.750000000000001,-2.44249065417534E-15,
3.78349364905421));
#370586=CARTESIAN_POINT('Ctrl Pts',(-0.750000000000001,0.433012701891373,
3.99999999999958));
#370587=CARTESIAN_POINT('Origin',(0.,2.73795905253904E-16,4.));
#370588=CARTESIAN_POINT('Origin',(0.,1.02673464470214E-16,4.));
#370589=CARTESIAN_POINT('',(-3.06161699786838E-16,2.5,4.));
#370590=CARTESIAN_POINT('Origin',(0.,1.02673464470214E-16,4.));
#370591=CARTESIAN_POINT('',(-3.06161699786838E-16,2.5,3.92500000000001));
#370592=CARTESIAN_POINT('',(-3.06161699786838E-16,2.5,4.));
#370593=CARTESIAN_POINT('Origin',(0.,9.75397912467035E-17,3.92500000000001));
#370594=CARTESIAN_POINT('Origin',(0.,9.75397912467035E-17,3.92500000000001));
#370595=CARTESIAN_POINT('',(-1.31649530908145E-16,1.0749999999984,2.49999999999841));
#370596=CARTESIAN_POINT('',(-3.06161699786838E-16,2.5,3.92500000000001));
#370597=CARTESIAN_POINT('',(-0.600917552801184,0.891360249694494,2.5));
#370598=CARTESIAN_POINT('Origin',(0.,0.,2.5));
#370599=CARTESIAN_POINT('Ctrl Pts',(1.21030729569027,-0.312499999998426,
2.67500000000005));
#370600=CARTESIAN_POINT('Ctrl Pts',(1.18496462782676,-0.397581898517953,
2.67173254198385));
#370601=CARTESIAN_POINT('Ctrl Pts',(1.15071194387983,-0.479744379279913,
2.66855106458315));
#370602=CARTESIAN_POINT('Ctrl Pts',(1.06411233511274,-0.63809170895112,
2.66237530137405));
#370603=CARTESIAN_POINT('Ctrl Pts',(1.01158452541921,-0.713299582901373,
2.6593557985417));
#370604=CARTESIAN_POINT('Ctrl Pts',(0.84399258075297,-0.902574391318878,
2.65021838828378));
#370605=CARTESIAN_POINT('Ctrl Pts',(0.71459255327479,-1.00055120699789,
2.643996728307));
#370606=CARTESIAN_POINT('Ctrl Pts',(0.434173163941591,-1.1360209702507,
2.63180275510934));
#370607=CARTESIAN_POINT('Ctrl Pts',(0.287439235068762,-1.17572689937217,
2.62594495039157));
#370608=CARTESIAN_POINT('Ctrl Pts',(-0.00405856185293136,-1.19866379085335,
2.61527944790127));
#370609=CARTESIAN_POINT('Ctrl Pts',(-0.161827341071919,-1.18631210777794,
2.61000562432497));
#370610=CARTESIAN_POINT('Ctrl Pts',(-0.469523736948815,-1.08498293735393,
2.59733204263689));
#370611=CARTESIAN_POINT('Ctrl Pts',(-0.603757024458315,-1.00920269685259,
2.59107878785054));
#370612=CARTESIAN_POINT('Ctrl Pts',(-0.861528187143977,-0.78774923249859,
2.57730651982981));
#370613=CARTESIAN_POINT('Ctrl Pts',(-0.949059710520787,-0.653224258938384,
2.57135243097231));
#370614=CARTESIAN_POINT('Ctrl Pts',(-1.06141710896073,-0.429890511860025,
2.56223771836896));
#370615=CARTESIAN_POINT('Ctrl Pts',(-1.09971742194718,-0.299695292969128,
2.55686044362927));
#370616=CARTESIAN_POINT('Ctrl Pts',(-1.12921272728689,-0.0226329958877538,
2.54523562102516));
#370617=CARTESIAN_POINT('Ctrl Pts',(-1.11665106720043,0.122177185089892,
2.53906054867293));
#370618=CARTESIAN_POINT('Ctrl Pts',(-1.03868521105767,0.394217153047777,
2.5272679762311));
#370619=CARTESIAN_POINT('Ctrl Pts',(-0.975394129424348,0.521041945584162,
2.52204255166252));
#370620=CARTESIAN_POINT('Ctrl Pts',(-0.810562892434841,0.735010845992019,
2.51135815914312));
#370621=CARTESIAN_POINT('Ctrl Pts',(-0.712460791732769,0.823114275812464,
2.50576422497663));
#370622=CARTESIAN_POINT('Ctrl Pts',(-0.600917552799552,0.891360249695952,
2.5000000000003));
#370623=CARTESIAN_POINT('',(0.93939647226611,-0.522646408087846,2.5));
#370624=CARTESIAN_POINT('Ctrl Pts',(0.939396472267503,-0.522646408088621,
2.49999999999841));
#370625=CARTESIAN_POINT('Ctrl Pts',(0.961378560063887,-0.493788939776118,
2.50517920331836));
#370626=CARTESIAN_POINT('Ctrl Pts',(0.981820055297906,-0.464129314934742,
2.51041697946993));
#370627=CARTESIAN_POINT('Ctrl Pts',(1.0007700635912,-0.433707147497555,
2.51570738971129));
#370628=CARTESIAN_POINT('Ctrl Pts',(1.01994614712023,-0.40292204097513,
2.52106091500378));
#370629=CARTESIAN_POINT('Ctrl Pts',(1.03759557945029,-0.37135536873159,
2.5264683377358));
#370630=CARTESIAN_POINT('Ctrl Pts',(1.05373251191938,-0.339009494244571,
2.53192350407058));
#370631=CARTESIAN_POINT('Ctrl Pts',(1.06650581336374,-0.313405891695234,
2.53624157903042));
#370632=CARTESIAN_POINT('Ctrl Pts',(1.07833079358038,-0.287313159438676,
2.54058956833869));
#370633=CARTESIAN_POINT('Ctrl Pts',(1.08919476231099,-0.260720293963244,
2.5449644199393));
#370634=CARTESIAN_POINT('Ctrl Pts',(1.10300386884231,-0.226918308571939,
2.55052525993339));
#370635=CARTESIAN_POINT('Ctrl Pts',(1.11523473813783,-0.192359407629985,
2.55612338880833));
#370636=CARTESIAN_POINT('Ctrl Pts',(1.12578644196984,-0.157280562137357,
2.56171996909941));
#370637=CARTESIAN_POINT('Ctrl Pts',(1.13631796415245,-0.122268809976041,
2.5673058451267));
#370638=CARTESIAN_POINT('Ctrl Pts',(1.14517642535264,-0.0867397266179055,
2.57289017848826));
#370639=CARTESIAN_POINT('Ctrl Pts',(1.15230846923948,-0.0509509669151141,
2.57843435414011));
#370640=CARTESIAN_POINT('Ctrl Pts',(1.15777287478455,-0.0235304546364063,
2.58268217210865));
#370641=CARTESIAN_POINT('Ctrl Pts',(1.16222477420995,0.00404196088120024,
2.58690641643057));
#370642=CARTESIAN_POINT('Ctrl Pts',(1.16566024779681,0.0316452258566077,
2.59108971936693));
#370643=CARTESIAN_POINT('Ctrl Pts',(1.16979235853104,0.0648458151264462,
2.59612130250411));
#370644=CARTESIAN_POINT('Ctrl Pts',(1.17249164294556,0.0984124738475194,
2.60114190384908));
#370645=CARTESIAN_POINT('Ctrl Pts',(1.17370841641877,0.132104984926701,
2.60611945789355));
#370646=CARTESIAN_POINT('Ctrl Pts',(1.17492748242562,0.16586097636351,2.61110639019154));
#370647=CARTESIAN_POINT('Ctrl Pts',(1.17465826041775,0.199742639149629,
2.61605011282462));
#370648=CARTESIAN_POINT('Ctrl Pts',(1.17290223392284,0.233497576361194,
2.62091837869804));
#370649=CARTESIAN_POINT('Ctrl Pts',(1.17114620742794,0.26725251357276,2.62578664457147));
#370650=CARTESIAN_POINT('Ctrl Pts',(1.16790337302496,0.300880045545673,
2.63057945368526));
#370651=CARTESIAN_POINT('Ctrl Pts',(1.16322801875488,0.334127040242341,
2.63526455894467));
#370652=CARTESIAN_POINT('Ctrl Pts',(1.1579563645548,0.371614393950363,2.6405472077862));
#370653=CARTESIAN_POINT('Ctrl Pts',(1.15086291017788,0.408718986722986,
2.64571065172927));
#370654=CARTESIAN_POINT('Ctrl Pts',(1.14196088119301,0.445439796657672,
2.65076150478858));
#370655=CARTESIAN_POINT('Ctrl Pts',(1.13310236418022,0.48198111999896,2.65578766992812));
#370656=CARTESIAN_POINT('Ctrl Pts',(1.12245275596893,0.518143424683796,
2.66070234215347));
#370657=CARTESIAN_POINT('Ctrl Pts',(1.10997435913185,0.553919706178163,
2.66551203896725));
#370658=CARTESIAN_POINT('Ctrl Pts',(1.1016495495542,0.577787414083731,2.66872076927321));
#370659=CARTESIAN_POINT('Ctrl Pts',(1.09250974434973,0.601483170784815,
2.67188277788132));
#370660=CARTESIAN_POINT('Ctrl Pts',(1.08253175473059,0.625000000000025,
2.67500000000006));
#370661=CARTESIAN_POINT('Origin',(0.,0.,2.5));
#370662=CARTESIAN_POINT('Origin',(-1.91190658769134E-30,5.47591810507809E-16,
4.));
#370663=CARTESIAN_POINT('',(-3.57786716920216E-15,0.866025403784441,4.));
#370664=CARTESIAN_POINT('Origin',(0.,2.73795905253904E-16,4.));
#370665=CARTESIAN_POINT('',(0.750000000000002,0.433012701892219,4.));
#370666=CARTESIAN_POINT('Origin',(0.,2.73795905253904E-16,4.));
#370667=CARTESIAN_POINT('',(0.750000000000002,-0.433012701892219,4.));
#370668=CARTESIAN_POINT('Origin',(0.,2.73795905253904E-16,4.));
#370669=CARTESIAN_POINT('',(-4.28259858131774E-15,-0.86602540378444,4.));
#370670=CARTESIAN_POINT('Origin',(0.,2.73795905253904E-16,4.));
#370671=CARTESIAN_POINT('Origin',(0.,2.73795905253904E-16,4.));
#370672=CARTESIAN_POINT('Origin',(-1.19494161730709E-30,3.4224488156738E-16,
2.5));
#370673=CARTESIAN_POINT('Ctrl Pts',(-0.600917552801664,0.891360249695444,
2.5));
#370674=CARTESIAN_POINT('Ctrl Pts',(-0.52912367055064,0.928118712066169,
2.5));
#370675=CARTESIAN_POINT('Ctrl Pts',(-0.45338281650616,0.956546033855086,
2.5));
#370676=CARTESIAN_POINT('Ctrl Pts',(-0.296173149603253,0.995821882185393,
2.5));
#370677=CARTESIAN_POINT('Ctrl Pts',(-0.215216702988762,1.00636894049577,
2.50000000001075));
#370678=CARTESIAN_POINT('Ctrl Pts',(-0.0605603584965276,1.00860738826189,
2.50000000001075));
#370679=CARTESIAN_POINT('Ctrl Pts',(0.0255986159637691,1.00270295342094,
2.5));
#370680=CARTESIAN_POINT('Ctrl Pts',(0.193358226390499,0.96153036876019,
2.5));
#370681=CARTESIAN_POINT('Ctrl Pts',(0.26576695744227,0.93389263995366,2.5));
#370682=CARTESIAN_POINT('Ctrl Pts',(0.333926106471282,0.897615791123228,
2.5));
#370683=CARTESIAN_POINT('Ctrl Pts',(0.870621065093339,0.39904851092642,
2.5));
#370684=CARTESIAN_POINT('Ctrl Pts',(0.912954540737191,0.330380547800277,
2.5));
#370685=CARTESIAN_POINT('Ctrl Pts',(0.946864699817239,0.256884680432555,
2.5));
#370686=CARTESIAN_POINT('Ctrl Pts',(0.996003967301862,0.104444769787427,
2.5));
#370687=CARTESIAN_POINT('Ctrl Pts',(1.01131329268253,0.0261625419559724,
2.5));
#370688=CARTESIAN_POINT('Ctrl Pts',(1.02292765596175,-0.129431544988595,
2.5));
#370689=CARTESIAN_POINT('Ctrl Pts',(1.01988149559102,-0.206142778785646,
2.5));
#370690=CARTESIAN_POINT('Ctrl Pts',(0.995349857534893,-0.364613759944385,
2.5));
#370691=CARTESIAN_POINT('Ctrl Pts',(0.972235069110387,-0.445515811209248,
2.5));
#370692=CARTESIAN_POINT('Ctrl Pts',(0.939396472266109,-0.522646408087845,
2.5));
#370693=CARTESIAN_POINT('Origin',(0.,2.73795905253904E-16,4.));
#370694=CARTESIAN_POINT('Ctrl Pts',(0.750000000000002,0.433012701891376,
3.99999999999958));
#370695=CARTESIAN_POINT('Ctrl Pts',(0.750000000000002,-4.71844785465692E-16,
3.78349364905421));
#370696=CARTESIAN_POINT('Ctrl Pts',(0.750000000000002,-0.433012701891378,
3.99999999999958));
#370697=CARTESIAN_POINT('Origin',(0.,2.73795905253904E-16,4.));
#370698=CARTESIAN_POINT('Ctrl Pts',(7.26431099148093E-13,0.866025403784019,
3.99999999999958));
#370699=CARTESIAN_POINT('Ctrl Pts',(0.375,0.649519052838329,3.78349364905421));
#370700=CARTESIAN_POINT('Ctrl Pts',(0.749999999999273,0.43301270189264,
3.99999999999958));
#370701=CARTESIAN_POINT('Origin',(0.,2.73795905253904E-16,4.));
#370702=CARTESIAN_POINT('Ctrl Pts',(-0.749999999999275,0.433012701892637,
3.99999999999958));
#370703=CARTESIAN_POINT('Ctrl Pts',(-0.375000000000002,0.649519052838327,
3.78349364905421));
#370704=CARTESIAN_POINT('Ctrl Pts',(-7.29620208486308E-13,0.866025403784017,
3.99999999999958));
#370705=CARTESIAN_POINT('Origin',(0.,2.73795905253904E-16,4.));
#370706=CARTESIAN_POINT('Ctrl Pts',(-7.33598022284514E-13,-0.866025403784019,
3.99999999999958));
#370707=CARTESIAN_POINT('Ctrl Pts',(-0.375000000000003,-0.649519052838331,
3.78349364905421));
#370708=CARTESIAN_POINT('Ctrl Pts',(-0.749999999999272,-0.433012701892644,
3.99999999999958));
#370709=CARTESIAN_POINT('Origin',(0.,2.73795905253904E-16,4.));
#370710=CARTESIAN_POINT('Ctrl Pts',(0.749999999999273,-0.433012701892642,
3.99999999999958));
#370711=CARTESIAN_POINT('Ctrl Pts',(0.375000000000001,-0.649519052838331,
3.78349364905421));
#370712=CARTESIAN_POINT('Ctrl Pts',(7.28385714548936E-13,-0.866025403784021,
3.99999999999958));
#370713=CARTESIAN_POINT('Origin',(0.750000000000002,-0.433012701892221,
2.95));
#370714=CARTESIAN_POINT('',(-8.98696932731E-16,-0.866025403784442,2.95));
#370715=CARTESIAN_POINT('',(0.750000000000002,-0.433012701892221,2.95));
#370716=CARTESIAN_POINT('',(-8.98696932731E-16,-0.866025403784442,2.95));
#370717=CARTESIAN_POINT('',(0.750000000000002,0.433012701892219,2.95));
#370718=CARTESIAN_POINT('',(0.750000000000002,-0.433012701892221,2.95));
#370719=CARTESIAN_POINT('',(6.5096847437113E-16,0.866025403784438,2.95));
#370720=CARTESIAN_POINT('',(0.750000000000002,0.433012701892219,2.95));
#370721=CARTESIAN_POINT('',(-0.750000000000001,0.433012701892218,2.95));
#370722=CARTESIAN_POINT('',(6.5096847437113E-16,0.866025403784438,2.95));
#370723=CARTESIAN_POINT('',(-0.750000000000001,-0.433012701892223,2.95));
#370724=CARTESIAN_POINT('',(-0.750000000000001,0.433012701892218,2.95));
#370725=CARTESIAN_POINT('',(-0.750000000000001,-0.433012701892223,2.95));
#370726=CARTESIAN_POINT('Origin',(0.750000000000002,-0.433012701892221,
2.95));
#370727=CARTESIAN_POINT('',(0.750000000000002,0.433012701892219,2.95));
#370728=CARTESIAN_POINT('',(0.750000000000002,-0.433012701892221,2.95));
#370729=CARTESIAN_POINT('Origin',(0.750000000000002,0.433012701892219,2.95));
#370730=CARTESIAN_POINT('',(6.5096847437113E-16,0.866025403784438,2.95));
#370731=CARTESIAN_POINT('Origin',(6.5096847437113E-16,0.866025403784438,
2.95));
#370732=CARTESIAN_POINT('',(-0.750000000000001,0.433012701892218,2.95));
#370733=CARTESIAN_POINT('Origin',(-0.750000000000001,0.433012701892218,
2.95));
#370734=CARTESIAN_POINT('',(-0.750000000000001,-0.433012701892223,2.95));
#370735=CARTESIAN_POINT('Origin',(-0.750000000000001,-0.433012701892223,
2.95));
#370736=CARTESIAN_POINT('',(-8.98696932731E-16,-0.866025403784442,2.95));
#370737=CARTESIAN_POINT('Origin',(-8.98696932731E-16,-0.866025403784442,
2.95));
#370738=CARTESIAN_POINT('Origin',(8.72870334710784E-15,-1.25,-4.00000000000001));
#370739=CARTESIAN_POINT('Ctrl Pts',(0.,0.957713005082983,-4.22499802480406));
#370740=CARTESIAN_POINT('Ctrl Pts',(-0.552935861291066,0.957713005082983,
-4.18749802480406));
#370741=CARTESIAN_POINT('Ctrl Pts',(-0.829403791936599,0.478856502541492,
-4.14999802480405));
#370742=CARTESIAN_POINT('Ctrl Pts',(-1.10587172258213,-6.632643158244E-17,
-4.11249802480406));
#370743=CARTESIAN_POINT('Ctrl Pts',(-0.829403791936599,-0.478856502541491,
-4.07499802480406));
#370744=CARTESIAN_POINT('Ctrl Pts',(-0.552935861291066,-0.957713005082983,
-4.03749802480406));
#370745=CARTESIAN_POINT('Ctrl Pts',(-1.17286016617667E-16,-0.957713005082983,
-3.99999802480406));
#370746=CARTESIAN_POINT('Ctrl Pts',(0.552935861291066,-0.957713005082984,
-3.96249802480406));
#370747=CARTESIAN_POINT('Ctrl Pts',(0.829403791936598,-0.478856502541492,
-3.92499802480406));
#370748=CARTESIAN_POINT('Ctrl Pts',(1.10587172258213,-3.36985585326162E-16,
-3.88749802480406));
#370749=CARTESIAN_POINT('Ctrl Pts',(0.829403791936599,0.478856502541491,
-3.84999802480406));
#370750=CARTESIAN_POINT('Ctrl Pts',(0.552935861291066,0.957713005082983,
-3.81249802480406));
#370751=CARTESIAN_POINT('Ctrl Pts',(0.,0.957713005082983,-3.77499802480406));
#370752=CARTESIAN_POINT('Ctrl Pts',(-0.552935861291066,0.957713005082983,
-3.73749802480406));
#370753=CARTESIAN_POINT('Ctrl Pts',(-0.829403791936599,0.478856502541492,
-3.69999802480406));
#370754=CARTESIAN_POINT('Ctrl Pts',(-1.10587172258213,-6.59238329387739E-17,
-3.66249802480405));
#370755=CARTESIAN_POINT('Ctrl Pts',(-0.829403791936599,-0.478856502541491,
-3.62499802480406));
#370756=CARTESIAN_POINT('Ctrl Pts',(-0.552935861291066,-0.957713005082983,
-3.58749802480406));
#370757=CARTESIAN_POINT('Ctrl Pts',(-1.17286016617667E-16,-0.957713005082983,
-3.54999802480406));
#370758=CARTESIAN_POINT('Ctrl Pts',(0.552935861291066,-0.957713005082984,
-3.51249802480406));
#370759=CARTESIAN_POINT('Ctrl Pts',(0.829403791936598,-0.478856502541492,
-3.47499802480406));
#370760=CARTESIAN_POINT('Ctrl Pts',(1.10587172258213,-3.36582986682496E-16,
-3.43749802480405));
#370761=CARTESIAN_POINT('Ctrl Pts',(0.829403791936599,0.478856502541491,
-3.39999802480406));
#370762=CARTESIAN_POINT('Ctrl Pts',(0.552935861291066,0.957713005082983,
-3.36249802480406));
#370763=CARTESIAN_POINT('Ctrl Pts',(0.,0.957713005082983,-3.32499802480406));
#370764=CARTESIAN_POINT('Ctrl Pts',(-0.552935861291066,0.957713005082983,
-3.28749802480406));
#370765=CARTESIAN_POINT('Ctrl Pts',(-0.829403791936599,0.478856502541492,
-3.24999802480406));
#370766=CARTESIAN_POINT('Ctrl Pts',(-1.10587172258213,-6.55212342951079E-17,
-3.21249802480406));
#370767=CARTESIAN_POINT('Ctrl Pts',(-0.829403791936599,-0.478856502541491,
-3.17499802480406));
#370768=CARTESIAN_POINT('Ctrl Pts',(-0.552935861291066,-0.957713005082983,
-3.13749802480406));
#370769=CARTESIAN_POINT('Ctrl Pts',(-1.17286016617667E-16,-0.957713005082983,
-3.09999802480406));
#370770=CARTESIAN_POINT('Ctrl Pts',(0.552935861291066,-0.957713005082984,
-3.06249802480406));
#370771=CARTESIAN_POINT('Ctrl Pts',(0.829403791936598,-0.478856502541492,
-3.02499802480406));
#370772=CARTESIAN_POINT('Ctrl Pts',(1.10587172258213,-3.3618038803883E-16,
-2.98749802480406));
#370773=CARTESIAN_POINT('Ctrl Pts',(0.829403791936599,0.478856502541491,
-2.94999802480406));
#370774=CARTESIAN_POINT('Ctrl Pts',(0.552935861291066,0.957713005082983,
-2.91249802480406));
#370775=CARTESIAN_POINT('Ctrl Pts',(0.,0.957713005082983,-2.87499802480406));
#370776=CARTESIAN_POINT('Ctrl Pts',(-0.552935861291066,0.957713005082983,
-2.83749802480406));
#370777=CARTESIAN_POINT('Ctrl Pts',(-0.829403791936599,0.478856502541492,
-2.79999802480406));
#370778=CARTESIAN_POINT('Ctrl Pts',(-1.10587172258213,-6.51186356514418E-17,
-2.76249802480406));
#370779=CARTESIAN_POINT('Ctrl Pts',(-0.829403791936599,-0.478856502541491,
-2.72499802480406));
#370780=CARTESIAN_POINT('Ctrl Pts',(-0.552935861291066,-0.957713005082983,
-2.68749802480406));
#370781=CARTESIAN_POINT('Ctrl Pts',(-1.17286016617667E-16,-0.957713005082983,
-2.64999802480406));
#370782=CARTESIAN_POINT('Ctrl Pts',(0.552935861291066,-0.957713005082984,
-2.61249802480406));
#370783=CARTESIAN_POINT('Ctrl Pts',(0.829403791936598,-0.478856502541492,
-2.57499802480406));
#370784=CARTESIAN_POINT('Ctrl Pts',(1.10587172258213,-3.35777789395164E-16,
-2.53749802480406));
#370785=CARTESIAN_POINT('Ctrl Pts',(0.829403791936599,0.478856502541491,
-2.49999802480406));
#370786=CARTESIAN_POINT('Ctrl Pts',(0.552935861291066,0.957713005082983,
-2.46249802480406));
#370787=CARTESIAN_POINT('Ctrl Pts',(0.,0.957713005082983,-2.42499802480406));
#370788=CARTESIAN_POINT('Ctrl Pts',(-0.552935861291066,0.957713005082983,
-2.38749802480406));
#370789=CARTESIAN_POINT('Ctrl Pts',(-0.829403791936599,0.478856502541492,
-2.34999802480406));
#370790=CARTESIAN_POINT('Ctrl Pts',(-1.10587172258213,-6.47160370077758E-17,
-2.31249802480406));
#370791=CARTESIAN_POINT('Ctrl Pts',(-0.829403791936599,-0.478856502541491,
-2.27499802480406));
#370792=CARTESIAN_POINT('Ctrl Pts',(-0.552935861291066,-0.957713005082983,
-2.23749802480406));
#370793=CARTESIAN_POINT('Ctrl Pts',(-1.17286016617667E-16,-0.957713005082983,
-2.19999802480406));
#370794=CARTESIAN_POINT('Ctrl Pts',(0.552935861291066,-0.957713005082984,
-2.16249802480406));
#370795=CARTESIAN_POINT('Ctrl Pts',(0.829403791936598,-0.478856502541492,
-2.12499802480406));
#370796=CARTESIAN_POINT('Ctrl Pts',(1.10587172258213,-3.35375190751498E-16,
-2.08749802480406));
#370797=CARTESIAN_POINT('Ctrl Pts',(0.829403791936599,0.478856502541491,
-2.04999802480406));
#370798=CARTESIAN_POINT('Ctrl Pts',(0.552935861291066,0.957713005082983,
-2.01249802480406));
#370799=CARTESIAN_POINT('Ctrl Pts',(0.,0.957713005082983,-1.97499802480406));
#370800=CARTESIAN_POINT('Ctrl Pts',(-0.552935861291066,0.957713005082983,
-1.93749802480406));
#370801=CARTESIAN_POINT('Ctrl Pts',(-0.829403791936599,0.478856502541492,
-1.89999802480406));
#370802=CARTESIAN_POINT('Ctrl Pts',(-1.10587172258213,-6.43134383641097E-17,
-1.86249802480406));
#370803=CARTESIAN_POINT('Ctrl Pts',(-0.829403791936599,-0.478856502541491,
-1.82499802480406));
#370804=CARTESIAN_POINT('Ctrl Pts',(-0.552935861291066,-0.957713005082983,
-1.78749802480406));
#370805=CARTESIAN_POINT('Ctrl Pts',(-1.17286016617667E-16,-0.957713005082983,
-1.74999802480406));
#370806=CARTESIAN_POINT('Ctrl Pts',(0.552935861291066,-0.957713005082984,
-1.71249802480406));
#370807=CARTESIAN_POINT('Ctrl Pts',(0.829403791936598,-0.478856502541492,
-1.67499802480406));
#370808=CARTESIAN_POINT('Ctrl Pts',(1.10587172258213,-3.34972592107832E-16,
-1.63749802480406));
#370809=CARTESIAN_POINT('Ctrl Pts',(0.829403791936599,0.478856502541491,
-1.59999802480406));
#370810=CARTESIAN_POINT('Ctrl Pts',(0.552935861291066,0.957713005082983,
-1.56249802480406));
#370811=CARTESIAN_POINT('Ctrl Pts',(0.,0.957713005082983,-1.52499802480406));
#370812=CARTESIAN_POINT('Ctrl Pts',(-0.552935861291066,0.957713005082983,
-1.48749802480406));
#370813=CARTESIAN_POINT('Ctrl Pts',(-0.829403791936599,0.478856502541492,
-1.44999802480406));
#370814=CARTESIAN_POINT('Ctrl Pts',(-1.10587172258213,-6.39108397204437E-17,
-1.41249802480406));
#370815=CARTESIAN_POINT('Ctrl Pts',(-0.829403791936599,-0.478856502541491,
-1.37499802480406));
#370816=CARTESIAN_POINT('Ctrl Pts',(-0.552935861291066,-0.957713005082983,
-1.33749802480406));
#370817=CARTESIAN_POINT('Ctrl Pts',(-1.17286016617667E-16,-0.957713005082983,
-1.29999802480406));
#370818=CARTESIAN_POINT('Ctrl Pts',(0.552935861291066,-0.957713005082984,
-1.26249802480406));
#370819=CARTESIAN_POINT('Ctrl Pts',(0.829403791936598,-0.478856502541492,
-1.22499802480406));
#370820=CARTESIAN_POINT('Ctrl Pts',(1.10587172258213,-3.34569993464166E-16,
-1.18749802480406));
#370821=CARTESIAN_POINT('Ctrl Pts',(0.829403791936599,0.478856502541491,
-1.14999802480406));
#370822=CARTESIAN_POINT('Ctrl Pts',(0.552935861291066,0.957713005082983,
-1.11249802480406));
#370823=CARTESIAN_POINT('Ctrl Pts',(0.,0.957713005082983,-1.07499802480406));
#370824=CARTESIAN_POINT('Ctrl Pts',(-0.552935861291066,0.957713005082983,
-1.03749802480406));
#370825=CARTESIAN_POINT('Ctrl Pts',(-0.829403791936599,0.478856502541492,
-0.999998024804056));
#370826=CARTESIAN_POINT('Ctrl Pts',(-1.10587172258213,-6.35082410767776E-17,
-0.962498024804056));
#370827=CARTESIAN_POINT('Ctrl Pts',(-0.829403791936599,-0.478856502541491,
-0.924998024804056));
#370828=CARTESIAN_POINT('Ctrl Pts',(-0.552935861291066,-0.957713005082983,
-0.887498024804056));
#370829=CARTESIAN_POINT('Ctrl Pts',(-1.17286016617667E-16,-0.957713005082983,
-0.849998024804056));
#370830=CARTESIAN_POINT('Ctrl Pts',(0.552935861291066,-0.957713005082984,
-0.812498024804056));
#370831=CARTESIAN_POINT('Ctrl Pts',(0.829403791936598,-0.478856502541492,
-0.774998024804056));
#370832=CARTESIAN_POINT('Ctrl Pts',(1.10587172258213,-3.341673948205E-16,
-0.737498024804056));
#370833=CARTESIAN_POINT('Ctrl Pts',(0.829403791936599,0.478856502541491,
-0.699998024804056));
#370834=CARTESIAN_POINT('Ctrl Pts',(0.552935861291066,0.957713005082983,
-0.662498024804056));
#370835=CARTESIAN_POINT('Ctrl Pts',(0.,0.957713005082983,-0.624998024804056));
#370836=CARTESIAN_POINT('Ctrl Pts',(-0.552935861291066,0.957713005082983,
-0.587498024804056));
#370837=CARTESIAN_POINT('Ctrl Pts',(-0.829403791936599,0.478856502541492,
-0.549998024804056));
#370838=CARTESIAN_POINT('Ctrl Pts',(-1.10587172258213,-6.31056424331116E-17,
-0.512498024804056));
#370839=CARTESIAN_POINT('Ctrl Pts',(-0.829403791936599,-0.478856502541491,
-0.474998024804056));
#370840=CARTESIAN_POINT('Ctrl Pts',(-0.552935861291066,-0.957713005082983,
-0.437498024804056));
#370841=CARTESIAN_POINT('Ctrl Pts',(-1.17286016617667E-16,-0.957713005082983,
-0.399998024804056));
#370842=CARTESIAN_POINT('Ctrl Pts',(0.552935861291066,-0.957713005082984,
-0.362498024804056));
#370843=CARTESIAN_POINT('Ctrl Pts',(0.829403791936598,-0.478856502541492,
-0.324998024804056));
#370844=CARTESIAN_POINT('Ctrl Pts',(1.10587172258213,-3.33764796176834E-16,
-0.287498024804056));
#370845=CARTESIAN_POINT('Ctrl Pts',(0.829403791936599,0.478856502541491,
-0.249998024804056));
#370846=CARTESIAN_POINT('Ctrl Pts',(0.552935861291066,0.957713005082983,
-0.212498024804056));
#370847=CARTESIAN_POINT('Ctrl Pts',(0.,0.957713005082983,-0.174998024804056));
#370848=CARTESIAN_POINT('Ctrl Pts',(-0.552935861291066,0.957713005082983,
-0.137498024804056));
#370849=CARTESIAN_POINT('Ctrl Pts',(-0.829403791936599,0.478856502541492,
-0.0999980248040564));
#370850=CARTESIAN_POINT('Ctrl Pts',(-1.10587172258213,-6.27030437894455E-17,
-0.0624980248040562));
#370851=CARTESIAN_POINT('Ctrl Pts',(-0.829403791936599,-0.478856502541491,
-0.024998024804056));
#370852=CARTESIAN_POINT('Ctrl Pts',(-0.552935861291066,-0.957713005082983,
0.0125019751959442));
#370853=CARTESIAN_POINT('Ctrl Pts',(-1.17286016617667E-16,-0.957713005082983,
0.0500019751959436));
#370854=CARTESIAN_POINT('Ctrl Pts',(0.552935861291066,-0.957713005082984,
0.0875019751959438));
#370855=CARTESIAN_POINT('Ctrl Pts',(0.829403791936598,-0.478856502541492,
0.125001975195944));
#370856=CARTESIAN_POINT('Ctrl Pts',(1.10587172258213,-3.33362197533168E-16,
0.162501975195944));
#370857=CARTESIAN_POINT('Ctrl Pts',(0.829403791936599,0.478856502541491,
0.200001975195944));
#370858=CARTESIAN_POINT('Ctrl Pts',(0.552935861291066,0.957713005082983,
0.237501975195944));
#370859=CARTESIAN_POINT('Ctrl Pts',(0.,0.957713005082983,0.275001975195944));
#370860=CARTESIAN_POINT('Ctrl Pts',(-0.552935861291066,0.957713005082983,
0.312501975195944));
#370861=CARTESIAN_POINT('Ctrl Pts',(-0.829403791936599,0.478856502541492,
0.350001975195944));
#370862=CARTESIAN_POINT('Ctrl Pts',(-1.10587172258213,-6.23004451457795E-17,
0.387501975195944));
#370863=CARTESIAN_POINT('Ctrl Pts',(-0.829403791936599,-0.478856502541491,
0.425001975195944));
#370864=CARTESIAN_POINT('Ctrl Pts',(-0.552935861291066,-0.957713005082983,
0.462501975195944));
#370865=CARTESIAN_POINT('Ctrl Pts',(-1.17286016617667E-16,-0.957713005082983,
0.500001975195943));
#370866=CARTESIAN_POINT('Ctrl Pts',(0.552935861291066,-0.957713005082984,
0.537501975195944));
#370867=CARTESIAN_POINT('Ctrl Pts',(0.829403791936598,-0.478856502541492,
0.575001975195944));
#370868=CARTESIAN_POINT('Ctrl Pts',(1.10587172258213,-3.32959598889502E-16,
0.612501975195944));
#370869=CARTESIAN_POINT('Ctrl Pts',(0.829403791936599,0.478856502541491,
0.650001975195944));
#370870=CARTESIAN_POINT('Ctrl Pts',(0.552935861291066,0.957713005082983,
0.687501975195943));
#370871=CARTESIAN_POINT('Ctrl Pts',(0.,0.957713005082983,0.725001975195944));
#370872=CARTESIAN_POINT('Ctrl Pts',(-0.552935861291066,0.957713005082983,
0.762501975195944));
#370873=CARTESIAN_POINT('Ctrl Pts',(-0.829403791936599,0.478856502541492,
0.800001975195944));
#370874=CARTESIAN_POINT('Ctrl Pts',(-1.10587172258213,-6.18978465021134E-17,
0.837501975195944));
#370875=CARTESIAN_POINT('Ctrl Pts',(-0.829403791936599,-0.478856502541491,
0.875001975195944));
#370876=CARTESIAN_POINT('Ctrl Pts',(-0.552935861291066,-0.957713005082983,
0.912501975195944));
#370877=CARTESIAN_POINT('Ctrl Pts',(-1.17286016617667E-16,-0.957713005082983,
0.950001975195944));
#370878=CARTESIAN_POINT('Ctrl Pts',(0.552935861291066,-0.957713005082984,
0.987501975195944));
#370879=CARTESIAN_POINT('Ctrl Pts',(0.829403791936598,-0.478856502541492,
1.02500197519594));
#370880=CARTESIAN_POINT('Ctrl Pts',(1.10587172258213,-3.32557000245836E-16,
1.06250197519594));
#370881=CARTESIAN_POINT('Ctrl Pts',(0.829403791936599,0.478856502541491,
1.10000197519594));
#370882=CARTESIAN_POINT('Ctrl Pts',(0.552935861291066,0.957713005082983,
1.13750197519594));
#370883=CARTESIAN_POINT('Ctrl Pts',(0.,0.957713005082983,1.17500197519594));
#370884=CARTESIAN_POINT('Ctrl Pts',(-0.552935861291066,0.957713005082983,
1.21250197519594));
#370885=CARTESIAN_POINT('Ctrl Pts',(-0.829403791936599,0.478856502541492,
1.25000197519594));
#370886=CARTESIAN_POINT('Ctrl Pts',(-1.10587172258213,-6.14952478584474E-17,
1.28750197519594));
#370887=CARTESIAN_POINT('Ctrl Pts',(-0.829403791936599,-0.478856502541491,
1.32500197519594));
#370888=CARTESIAN_POINT('Ctrl Pts',(-0.552935861291066,-0.957713005082983,
1.36250197519594));
#370889=CARTESIAN_POINT('Ctrl Pts',(-1.17286016617667E-16,-0.957713005082983,
1.40000197519594));
#370890=CARTESIAN_POINT('Ctrl Pts',(0.552935861291066,-0.957713005082984,
1.43750197519594));
#370891=CARTESIAN_POINT('Ctrl Pts',(0.829403791936598,-0.478856502541492,
1.47500197519594));
#370892=CARTESIAN_POINT('Ctrl Pts',(1.10587172258213,-3.3215440160217E-16,
1.51250197519594));
#370893=CARTESIAN_POINT('Ctrl Pts',(0.829403791936599,0.478856502541491,
1.55000197519594));
#370894=CARTESIAN_POINT('Ctrl Pts',(0.552935861291066,0.957713005082983,
1.58750197519594));
#370895=CARTESIAN_POINT('Ctrl Pts',(0.,0.957713005082983,1.62500197519594));
#370896=CARTESIAN_POINT('Ctrl Pts',(-0.552935861291066,0.957713005082983,
1.66250197519594));
#370897=CARTESIAN_POINT('Ctrl Pts',(-0.829403791936599,0.478856502541492,
1.70000197519594));
#370898=CARTESIAN_POINT('Ctrl Pts',(-1.10587172258213,-6.10926492147814E-17,
1.73750197519594));
#370899=CARTESIAN_POINT('Ctrl Pts',(-0.829403791936599,-0.478856502541491,
1.77500197519594));
#370900=CARTESIAN_POINT('Ctrl Pts',(-0.552935861291066,-0.957713005082983,
1.81250197519594));
#370901=CARTESIAN_POINT('Ctrl Pts',(-1.17286016617667E-16,-0.957713005082983,
1.85000197519594));
#370902=CARTESIAN_POINT('Ctrl Pts',(0.552935861291066,-0.957713005082984,
1.88750197519594));
#370903=CARTESIAN_POINT('Ctrl Pts',(0.829403791936598,-0.478856502541492,
1.92500197519594));
#370904=CARTESIAN_POINT('Ctrl Pts',(1.10587172258213,-3.31751802958504E-16,
1.96250197519594));
#370905=CARTESIAN_POINT('Ctrl Pts',(0.829403791936599,0.478856502541491,
2.00000197519594));
#370906=CARTESIAN_POINT('Ctrl Pts',(0.552935861291066,0.957713005082983,
2.03750197519594));
#370907=CARTESIAN_POINT('Ctrl Pts',(0.,0.957713005082983,2.07500197519594));
#370908=CARTESIAN_POINT('Ctrl Pts',(-0.552935861291066,0.957713005082983,
2.11250197519594));
#370909=CARTESIAN_POINT('Ctrl Pts',(-0.829403791936599,0.478856502541492,
2.15000197519594));
#370910=CARTESIAN_POINT('Ctrl Pts',(-1.10587172258213,-6.06900505711153E-17,
2.18750197519594));
#370911=CARTESIAN_POINT('Ctrl Pts',(-0.829403791936599,-0.478856502541491,
2.22500197519594));
#370912=CARTESIAN_POINT('Ctrl Pts',(-0.552935861291066,-0.957713005082983,
2.26250197519594));
#370913=CARTESIAN_POINT('Ctrl Pts',(-1.17286016617667E-16,-0.957713005082983,
2.30000197519594));
#370914=CARTESIAN_POINT('Ctrl Pts',(0.552935861291066,-0.957713005082984,
2.33750197519594));
#370915=CARTESIAN_POINT('Ctrl Pts',(0.829403791936598,-0.478856502541492,
2.37500197519594));
#370916=CARTESIAN_POINT('Ctrl Pts',(1.10587172258213,-3.31349204314838E-16,
2.41250197519594));
#370917=CARTESIAN_POINT('Ctrl Pts',(0.829403791936599,0.478856502541491,
2.45000197519594));
#370918=CARTESIAN_POINT('Ctrl Pts',(0.552935861291066,0.957713005082983,
2.48750197519594));
#370919=CARTESIAN_POINT('Ctrl Pts',(0.,0.957713005082983,2.52500197519594));
#370920=CARTESIAN_POINT('Ctrl Pts',(-0.552935861291066,0.957713005082983,
2.56250197519594));
#370921=CARTESIAN_POINT('Ctrl Pts',(-0.829403791936599,0.478856502541492,
2.60000197519594));
#370922=CARTESIAN_POINT('Ctrl Pts',(-1.10587172258213,-6.02874519274493E-17,
2.63750197519594));
#370923=CARTESIAN_POINT('Ctrl Pts',(-0.829403791936599,-0.478856502541491,
2.67500197519594));
#370924=CARTESIAN_POINT('Ctrl Pts',(-0.552935861291066,-0.957713005082983,
2.71250197519594));
#370925=CARTESIAN_POINT('Ctrl Pts',(-1.17286016617667E-16,-0.957713005082983,
2.75000197519594));
#370926=CARTESIAN_POINT('Ctrl Pts',(0.552935861291066,-0.957713005082984,
2.78750197519594));
#370927=CARTESIAN_POINT('Ctrl Pts',(0.829403791936598,-0.478856502541492,
2.82500197519594));
#370928=CARTESIAN_POINT('Ctrl Pts',(1.10587172258213,-3.30946605671172E-16,
2.86250197519594));
#370929=CARTESIAN_POINT('Ctrl Pts',(0.829403791936599,0.478856502541491,
2.90000197519594));
#370930=CARTESIAN_POINT('Ctrl Pts',(0.552935861291066,0.957713005082983,
2.93750197519594));
#370931=CARTESIAN_POINT('Ctrl Pts',(0.,0.957713005082983,2.97500197519594));
#370932=CARTESIAN_POINT('Ctrl Pts',(-0.552935861291066,0.957713005082983,
3.01250197519594));
#370933=CARTESIAN_POINT('Ctrl Pts',(-0.829403791936599,0.478856502541492,
3.05000197519594));
#370934=CARTESIAN_POINT('Ctrl Pts',(-1.10587172258213,-5.98848532837832E-17,
3.08750197519594));
#370935=CARTESIAN_POINT('Ctrl Pts',(-0.829403791936599,-0.478856502541491,
3.12500197519594));
#370936=CARTESIAN_POINT('Ctrl Pts',(-0.552935861291066,-0.957713005082983,
3.16250197519594));
#370937=CARTESIAN_POINT('Ctrl Pts',(-1.17286016617667E-16,-0.957713005082983,
3.20000197519594));
#370938=CARTESIAN_POINT('Ctrl Pts',(0.552935861291066,-0.957713005082984,
3.23750197519594));
#370939=CARTESIAN_POINT('Ctrl Pts',(0.829403791936598,-0.478856502541492,
3.27500197519594));
#370940=CARTESIAN_POINT('Ctrl Pts',(1.10587172258213,-3.30544007027506E-16,
3.31250197519594));
#370941=CARTESIAN_POINT('Ctrl Pts',(0.829403791936599,0.478856502541491,
3.35000197519594));
#370942=CARTESIAN_POINT('Ctrl Pts',(0.552935861291066,0.957713005082983,
3.38750197519594));
#370943=CARTESIAN_POINT('Ctrl Pts',(0.,0.957713005082983,3.42500197519594));
#370944=CARTESIAN_POINT('Ctrl Pts',(-0.552935861291066,0.957713005082983,
3.46250197519594));
#370945=CARTESIAN_POINT('Ctrl Pts',(-0.829403791936599,0.478856502541492,
3.50000197519594));
#370946=CARTESIAN_POINT('Ctrl Pts',(-1.10587172258213,-5.94822546401172E-17,
3.53750197519594));
#370947=CARTESIAN_POINT('Ctrl Pts',(-0.829403791936599,-0.478856502541491,
3.57500197519594));
#370948=CARTESIAN_POINT('Ctrl Pts',(-0.552935861291066,-0.957713005082983,
3.61250197519594));
#370949=CARTESIAN_POINT('Ctrl Pts',(-1.17286016617667E-16,-0.957713005082983,
3.65000197519594));
#370950=CARTESIAN_POINT('Ctrl Pts',(0.552935861291066,-0.957713005082984,
3.68750197519594));
#370951=CARTESIAN_POINT('Ctrl Pts',(0.829403791936598,-0.478856502541492,
3.72500197519594));
#370952=CARTESIAN_POINT('Ctrl Pts',(1.0036847708126,-0.176992992335418,
3.74864137775736));
#370953=CARTESIAN_POINT('Ctrl Pts',(0.943168426706962,0.166275431041969,
3.77552326368421));
#370954=CARTESIAN_POINT('Ctrl Pts',(0.848846015356109,0.701302883742039,
3.81742209844946));
#370955=CARTESIAN_POINT('Ctrl Pts',(0.754523604005256,1.23633033644211,
3.85932093321471));
#370956=CARTESIAN_POINT('Ctrl Pts',(0.,1.27435696448144,-4.40781250000002));
#370957=CARTESIAN_POINT('Ctrl Pts',(-0.735750336487031,1.27435696448144,
-4.37031250000002));
#370958=CARTESIAN_POINT('Ctrl Pts',(-1.10362550473055,0.637178482240718,
-4.33281250000002));
#370959=CARTESIAN_POINT('Ctrl Pts',(-1.47150067297406,-4.41016728599111E-17,
-4.29531250000002));
#370960=CARTESIAN_POINT('Ctrl Pts',(-1.10362550473055,-0.637178482240718,
-4.25781250000002));
#370961=CARTESIAN_POINT('Ctrl Pts',(-0.735750336487032,-1.27435696448144,
-4.22031250000002));
#370962=CARTESIAN_POINT('Ctrl Pts',(-1.56063717752333E-16,-1.27435696448144,
-4.18281250000002));
#370963=CARTESIAN_POINT('Ctrl Pts',(0.735750336487031,-1.27435696448144,
-4.14531250000002));
#370964=CARTESIAN_POINT('Ctrl Pts',(1.10362550473055,-0.637178482240719,
-4.10781250000002));
#370965=CARTESIAN_POINT('Ctrl Pts',(1.47150067297406,-4.0431409135825E-16,
-4.07031250000002));
#370966=CARTESIAN_POINT('Ctrl Pts',(1.10362550473055,0.637178482240717,
-4.03281250000002));
#370967=CARTESIAN_POINT('Ctrl Pts',(0.735750336487032,1.27435696448144,
-3.99531250000002));
#370968=CARTESIAN_POINT('Ctrl Pts',(0.,1.27435696448144,-3.95781250000002));
#370969=CARTESIAN_POINT('Ctrl Pts',(-0.735750336487031,1.27435696448144,
-3.92031250000002));
#370970=CARTESIAN_POINT('Ctrl Pts',(-1.10362550473055,0.637178482240718,
-3.88281250000002));
#370971=CARTESIAN_POINT('Ctrl Pts',(-1.47150067297406,-4.3699074216245E-17,
-3.84531250000002));
#370972=CARTESIAN_POINT('Ctrl Pts',(-1.10362550473055,-0.637178482240718,
-3.80781250000002));
#370973=CARTESIAN_POINT('Ctrl Pts',(-0.735750336487032,-1.27435696448144,
-3.77031250000002));
#370974=CARTESIAN_POINT('Ctrl Pts',(-1.56063717752333E-16,-1.27435696448144,
-3.73281250000002));
#370975=CARTESIAN_POINT('Ctrl Pts',(0.735750336487031,-1.27435696448144,
-3.69531250000002));
#370976=CARTESIAN_POINT('Ctrl Pts',(1.10362550473055,-0.637178482240719,
-3.65781250000002));
#370977=CARTESIAN_POINT('Ctrl Pts',(1.47150067297406,-4.03911492714584E-16,
-3.62031250000002));
#370978=CARTESIAN_POINT('Ctrl Pts',(1.10362550473055,0.637178482240717,
-3.58281250000002));
#370979=CARTESIAN_POINT('Ctrl Pts',(0.735750336487032,1.27435696448144,
-3.54531250000002));
#370980=CARTESIAN_POINT('Ctrl Pts',(0.,1.27435696448144,-3.50781250000002));
#370981=CARTESIAN_POINT('Ctrl Pts',(-0.735750336487031,1.27435696448144,
-3.47031250000002));
#370982=CARTESIAN_POINT('Ctrl Pts',(-1.10362550473055,0.637178482240718,
-3.43281250000002));
#370983=CARTESIAN_POINT('Ctrl Pts',(-1.47150067297406,-4.3296475572579E-17,
-3.39531250000002));
#370984=CARTESIAN_POINT('Ctrl Pts',(-1.10362550473055,-0.637178482240718,
-3.35781250000002));
#370985=CARTESIAN_POINT('Ctrl Pts',(-0.735750336487032,-1.27435696448144,
-3.32031250000002));
#370986=CARTESIAN_POINT('Ctrl Pts',(-1.56063717752333E-16,-1.27435696448144,
-3.28281250000002));
#370987=CARTESIAN_POINT('Ctrl Pts',(0.735750336487031,-1.27435696448144,
-3.24531250000002));
#370988=CARTESIAN_POINT('Ctrl Pts',(1.10362550473055,-0.637178482240719,
-3.20781250000002));
#370989=CARTESIAN_POINT('Ctrl Pts',(1.47150067297406,-4.03508894070918E-16,
-3.17031250000002));
#370990=CARTESIAN_POINT('Ctrl Pts',(1.10362550473055,0.637178482240717,
-3.13281250000002));
#370991=CARTESIAN_POINT('Ctrl Pts',(0.735750336487032,1.27435696448144,
-3.09531250000002));
#370992=CARTESIAN_POINT('Ctrl Pts',(0.,1.27435696448144,-3.05781250000002));
#370993=CARTESIAN_POINT('Ctrl Pts',(-0.735750336487031,1.27435696448144,
-3.02031250000002));
#370994=CARTESIAN_POINT('Ctrl Pts',(-1.10362550473055,0.637178482240718,
-2.98281250000002));
#370995=CARTESIAN_POINT('Ctrl Pts',(-1.47150067297406,-4.28938769289129E-17,
-2.94531250000002));
#370996=CARTESIAN_POINT('Ctrl Pts',(-1.10362550473055,-0.637178482240718,
-2.90781250000002));
#370997=CARTESIAN_POINT('Ctrl Pts',(-0.735750336487032,-1.27435696448144,
-2.87031250000002));
#370998=CARTESIAN_POINT('Ctrl Pts',(-1.56063717752333E-16,-1.27435696448144,
-2.83281250000002));
#370999=CARTESIAN_POINT('Ctrl Pts',(0.735750336487031,-1.27435696448144,
-2.79531250000002));
#371000=CARTESIAN_POINT('Ctrl Pts',(1.10362550473055,-0.637178482240719,
-2.75781250000002));
#371001=CARTESIAN_POINT('Ctrl Pts',(1.47150067297406,-4.03106295427252E-16,
-2.72031250000002));
#371002=CARTESIAN_POINT('Ctrl Pts',(1.10362550473055,0.637178482240717,
-2.68281250000002));
#371003=CARTESIAN_POINT('Ctrl Pts',(0.735750336487032,1.27435696448144,
-2.64531250000002));
#371004=CARTESIAN_POINT('Ctrl Pts',(0.,1.27435696448144,-2.60781250000002));
#371005=CARTESIAN_POINT('Ctrl Pts',(-0.735750336487031,1.27435696448144,
-2.57031250000002));
#371006=CARTESIAN_POINT('Ctrl Pts',(-1.10362550473055,0.637178482240718,
-2.53281250000002));
#371007=CARTESIAN_POINT('Ctrl Pts',(-1.47150067297406,-4.24912782852469E-17,
-2.49531250000002));
#371008=CARTESIAN_POINT('Ctrl Pts',(-1.10362550473055,-0.637178482240718,
-2.45781250000002));
#371009=CARTESIAN_POINT('Ctrl Pts',(-0.735750336487032,-1.27435696448144,
-2.42031250000002));
#371010=CARTESIAN_POINT('Ctrl Pts',(-1.56063717752333E-16,-1.27435696448144,
-2.38281250000002));
#371011=CARTESIAN_POINT('Ctrl Pts',(0.735750336487031,-1.27435696448144,
-2.34531250000002));
#371012=CARTESIAN_POINT('Ctrl Pts',(1.10362550473055,-0.637178482240719,
-2.30781250000002));
#371013=CARTESIAN_POINT('Ctrl Pts',(1.47150067297406,-4.02703696783586E-16,
-2.27031250000002));
#371014=CARTESIAN_POINT('Ctrl Pts',(1.10362550473055,0.637178482240717,
-2.23281250000002));
#371015=CARTESIAN_POINT('Ctrl Pts',(0.735750336487032,1.27435696448144,
-2.19531250000002));
#371016=CARTESIAN_POINT('Ctrl Pts',(0.,1.27435696448144,-2.15781250000002));
#371017=CARTESIAN_POINT('Ctrl Pts',(-0.735750336487031,1.27435696448144,
-2.12031250000002));
#371018=CARTESIAN_POINT('Ctrl Pts',(-1.10362550473055,0.637178482240718,
-2.08281250000002));
#371019=CARTESIAN_POINT('Ctrl Pts',(-1.47150067297406,-4.20886796415808E-17,
-2.04531250000002));
#371020=CARTESIAN_POINT('Ctrl Pts',(-1.10362550473055,-0.637178482240718,
-2.00781250000002));
#371021=CARTESIAN_POINT('Ctrl Pts',(-0.735750336487032,-1.27435696448144,
-1.97031250000002));
#371022=CARTESIAN_POINT('Ctrl Pts',(-1.56063717752333E-16,-1.27435696448144,
-1.93281250000002));
#371023=CARTESIAN_POINT('Ctrl Pts',(0.735750336487031,-1.27435696448144,
-1.89531250000002));
#371024=CARTESIAN_POINT('Ctrl Pts',(1.10362550473055,-0.637178482240719,
-1.85781250000002));
#371025=CARTESIAN_POINT('Ctrl Pts',(1.47150067297406,-4.0230109813992E-16,
-1.82031250000002));
#371026=CARTESIAN_POINT('Ctrl Pts',(1.10362550473055,0.637178482240717,
-1.78281250000002));
#371027=CARTESIAN_POINT('Ctrl Pts',(0.735750336487032,1.27435696448144,
-1.74531250000002));
#371028=CARTESIAN_POINT('Ctrl Pts',(0.,1.27435696448144,-1.70781250000002));
#371029=CARTESIAN_POINT('Ctrl Pts',(-0.735750336487031,1.27435696448144,
-1.67031250000002));
#371030=CARTESIAN_POINT('Ctrl Pts',(-1.10362550473055,0.637178482240718,
-1.63281250000002));
#371031=CARTESIAN_POINT('Ctrl Pts',(-1.47150067297406,-4.16860809979148E-17,
-1.59531250000002));
#371032=CARTESIAN_POINT('Ctrl Pts',(-1.10362550473055,-0.637178482240718,
-1.55781250000002));
#371033=CARTESIAN_POINT('Ctrl Pts',(-0.735750336487032,-1.27435696448144,
-1.52031250000002));
#371034=CARTESIAN_POINT('Ctrl Pts',(-1.56063717752333E-16,-1.27435696448144,
-1.48281250000002));
#371035=CARTESIAN_POINT('Ctrl Pts',(0.735750336487031,-1.27435696448144,
-1.44531250000002));
#371036=CARTESIAN_POINT('Ctrl Pts',(1.10362550473055,-0.637178482240719,
-1.40781250000002));
#371037=CARTESIAN_POINT('Ctrl Pts',(1.47150067297406,-4.01898499496254E-16,
-1.37031250000002));
#371038=CARTESIAN_POINT('Ctrl Pts',(1.10362550473055,0.637178482240717,
-1.33281250000002));
#371039=CARTESIAN_POINT('Ctrl Pts',(0.735750336487032,1.27435696448144,
-1.29531250000002));
#371040=CARTESIAN_POINT('Ctrl Pts',(0.,1.27435696448144,-1.25781250000002));
#371041=CARTESIAN_POINT('Ctrl Pts',(-0.735750336487031,1.27435696448144,
-1.22031250000002));
#371042=CARTESIAN_POINT('Ctrl Pts',(-1.10362550473055,0.637178482240718,
-1.18281250000002));
#371043=CARTESIAN_POINT('Ctrl Pts',(-1.47150067297406,-4.12834823542487E-17,
-1.14531250000002));
#371044=CARTESIAN_POINT('Ctrl Pts',(-1.10362550473055,-0.637178482240718,
-1.10781250000002));
#371045=CARTESIAN_POINT('Ctrl Pts',(-0.735750336487032,-1.27435696448144,
-1.07031250000002));
#371046=CARTESIAN_POINT('Ctrl Pts',(-1.56063717752333E-16,-1.27435696448144,
-1.03281250000002));
#371047=CARTESIAN_POINT('Ctrl Pts',(0.735750336487031,-1.27435696448144,
-0.995312500000018));
#371048=CARTESIAN_POINT('Ctrl Pts',(1.10362550473055,-0.637178482240719,
-0.957812500000018));
#371049=CARTESIAN_POINT('Ctrl Pts',(1.47150067297406,-4.01495900852588E-16,
-0.920312500000018));
#371050=CARTESIAN_POINT('Ctrl Pts',(1.10362550473055,0.637178482240717,
-0.882812500000018));
#371051=CARTESIAN_POINT('Ctrl Pts',(0.735750336487032,1.27435696448144,
-0.845312500000018));
#371052=CARTESIAN_POINT('Ctrl Pts',(0.,1.27435696448144,-0.807812500000018));
#371053=CARTESIAN_POINT('Ctrl Pts',(-0.735750336487031,1.27435696448144,
-0.770312500000018));
#371054=CARTESIAN_POINT('Ctrl Pts',(-1.10362550473055,0.637178482240718,
-0.732812500000018));
#371055=CARTESIAN_POINT('Ctrl Pts',(-1.47150067297406,-4.08808837105827E-17,
-0.695312500000018));
#371056=CARTESIAN_POINT('Ctrl Pts',(-1.10362550473055,-0.637178482240718,
-0.657812500000018));
#371057=CARTESIAN_POINT('Ctrl Pts',(-0.735750336487032,-1.27435696448144,
-0.620312500000018));
#371058=CARTESIAN_POINT('Ctrl Pts',(-1.56063717752333E-16,-1.27435696448144,
-0.582812500000018));
#371059=CARTESIAN_POINT('Ctrl Pts',(0.735750336487031,-1.27435696448144,
-0.545312500000018));
#371060=CARTESIAN_POINT('Ctrl Pts',(1.10362550473055,-0.637178482240719,
-0.507812500000018));
#371061=CARTESIAN_POINT('Ctrl Pts',(1.47150067297406,-4.01093302208922E-16,
-0.470312500000018));
#371062=CARTESIAN_POINT('Ctrl Pts',(1.10362550473055,0.637178482240717,
-0.432812500000018));
#371063=CARTESIAN_POINT('Ctrl Pts',(0.735750336487032,1.27435696448144,
-0.395312500000018));
#371064=CARTESIAN_POINT('Ctrl Pts',(0.,1.27435696448144,-0.357812500000018));
#371065=CARTESIAN_POINT('Ctrl Pts',(-0.735750336487031,1.27435696448144,
-0.320312500000018));
#371066=CARTESIAN_POINT('Ctrl Pts',(-1.10362550473055,0.637178482240718,
-0.282812500000018));
#371067=CARTESIAN_POINT('Ctrl Pts',(-1.47150067297406,-4.04782850669166E-17,
-0.245312500000018));
#371068=CARTESIAN_POINT('Ctrl Pts',(-1.10362550473055,-0.637178482240718,
-0.207812500000018));
#371069=CARTESIAN_POINT('Ctrl Pts',(-0.735750336487032,-1.27435696448144,
-0.170312500000018));
#371070=CARTESIAN_POINT('Ctrl Pts',(-1.56063717752333E-16,-1.27435696448144,
-0.132812500000018));
#371071=CARTESIAN_POINT('Ctrl Pts',(0.735750336487031,-1.27435696448144,
-0.0953125000000181));
#371072=CARTESIAN_POINT('Ctrl Pts',(1.10362550473055,-0.637178482240719,
-0.0578125000000179));
#371073=CARTESIAN_POINT('Ctrl Pts',(1.47150067297406,-4.00690703565256E-16,
-0.0203125000000177));
#371074=CARTESIAN_POINT('Ctrl Pts',(1.10362550473055,0.637178482240717,
0.0171874999999816));
#371075=CARTESIAN_POINT('Ctrl Pts',(0.735750336487032,1.27435696448144,
0.0546874999999818));
#371076=CARTESIAN_POINT('Ctrl Pts',(0.,1.27435696448144,0.0921874999999821));
#371077=CARTESIAN_POINT('Ctrl Pts',(-0.735750336487031,1.27435696448144,
0.129687499999982));
#371078=CARTESIAN_POINT('Ctrl Pts',(-1.10362550473055,0.637178482240718,
0.167187499999982));
#371079=CARTESIAN_POINT('Ctrl Pts',(-1.47150067297406,-4.00756864232506E-17,
0.204687499999982));
#371080=CARTESIAN_POINT('Ctrl Pts',(-1.10362550473055,-0.637178482240718,
0.242187499999982));
#371081=CARTESIAN_POINT('Ctrl Pts',(-0.735750336487032,-1.27435696448144,
0.279687499999982));
#371082=CARTESIAN_POINT('Ctrl Pts',(-1.56063717752333E-16,-1.27435696448144,
0.317187499999982));
#371083=CARTESIAN_POINT('Ctrl Pts',(0.735750336487031,-1.27435696448144,
0.354687499999982));
#371084=CARTESIAN_POINT('Ctrl Pts',(1.10362550473055,-0.637178482240719,
0.392187499999982));
#371085=CARTESIAN_POINT('Ctrl Pts',(1.47150067297406,-4.0028810492159E-16,
0.429687499999982));
#371086=CARTESIAN_POINT('Ctrl Pts',(1.10362550473055,0.637178482240717,
0.467187499999982));
#371087=CARTESIAN_POINT('Ctrl Pts',(0.735750336487032,1.27435696448144,
0.504687499999982));
#371088=CARTESIAN_POINT('Ctrl Pts',(0.,1.27435696448144,0.542187499999982));
#371089=CARTESIAN_POINT('Ctrl Pts',(-0.735750336487031,1.27435696448144,
0.579687499999982));
#371090=CARTESIAN_POINT('Ctrl Pts',(-1.10362550473055,0.637178482240718,
0.617187499999982));
#371091=CARTESIAN_POINT('Ctrl Pts',(-1.47150067297406,-3.96730877795845E-17,
0.654687499999982));
#371092=CARTESIAN_POINT('Ctrl Pts',(-1.10362550473055,-0.637178482240718,
0.692187499999982));
#371093=CARTESIAN_POINT('Ctrl Pts',(-0.735750336487032,-1.27435696448144,
0.729687499999982));
#371094=CARTESIAN_POINT('Ctrl Pts',(-1.56063717752333E-16,-1.27435696448144,
0.767187499999982));
#371095=CARTESIAN_POINT('Ctrl Pts',(0.735750336487031,-1.27435696448144,
0.804687499999982));
#371096=CARTESIAN_POINT('Ctrl Pts',(1.10362550473055,-0.637178482240719,
0.842187499999982));
#371097=CARTESIAN_POINT('Ctrl Pts',(1.47150067297406,-3.99885506277924E-16,
0.879687499999982));
#371098=CARTESIAN_POINT('Ctrl Pts',(1.10362550473055,0.637178482240717,
0.917187499999982));
#371099=CARTESIAN_POINT('Ctrl Pts',(0.735750336487032,1.27435696448144,
0.954687499999982));
#371100=CARTESIAN_POINT('Ctrl Pts',(0.,1.27435696448144,0.992187499999982));
#371101=CARTESIAN_POINT('Ctrl Pts',(-0.735750336487031,1.27435696448144,
1.02968749999998));
#371102=CARTESIAN_POINT('Ctrl Pts',(-1.10362550473055,0.637178482240718,
1.06718749999998));
#371103=CARTESIAN_POINT('Ctrl Pts',(-1.47150067297406,-3.92704891359185E-17,
1.10468749999998));
#371104=CARTESIAN_POINT('Ctrl Pts',(-1.10362550473055,-0.637178482240718,
1.14218749999998));
#371105=CARTESIAN_POINT('Ctrl Pts',(-0.735750336487032,-1.27435696448144,
1.17968749999998));
#371106=CARTESIAN_POINT('Ctrl Pts',(-1.56063717752333E-16,-1.27435696448144,
1.21718749999998));
#371107=CARTESIAN_POINT('Ctrl Pts',(0.735750336487031,-1.27435696448144,
1.25468749999998));
#371108=CARTESIAN_POINT('Ctrl Pts',(1.10362550473055,-0.637178482240719,
1.29218749999998));
#371109=CARTESIAN_POINT('Ctrl Pts',(1.47150067297406,-3.99482907634258E-16,
1.32968749999998));
#371110=CARTESIAN_POINT('Ctrl Pts',(1.10362550473055,0.637178482240717,
1.36718749999998));
#371111=CARTESIAN_POINT('Ctrl Pts',(0.735750336487032,1.27435696448144,
1.40468749999998));
#371112=CARTESIAN_POINT('Ctrl Pts',(0.,1.27435696448144,1.44218749999998));
#371113=CARTESIAN_POINT('Ctrl Pts',(-0.735750336487031,1.27435696448144,
1.47968749999998));
#371114=CARTESIAN_POINT('Ctrl Pts',(-1.10362550473055,0.637178482240718,
1.51718749999998));
#371115=CARTESIAN_POINT('Ctrl Pts',(-1.47150067297406,-3.88678904922525E-17,
1.55468749999998));
#371116=CARTESIAN_POINT('Ctrl Pts',(-1.10362550473055,-0.637178482240718,
1.59218749999998));
#371117=CARTESIAN_POINT('Ctrl Pts',(-0.735750336487032,-1.27435696448144,
1.62968749999998));
#371118=CARTESIAN_POINT('Ctrl Pts',(-1.56063717752333E-16,-1.27435696448144,
1.66718749999998));
#371119=CARTESIAN_POINT('Ctrl Pts',(0.735750336487031,-1.27435696448144,
1.70468749999998));
#371120=CARTESIAN_POINT('Ctrl Pts',(1.10362550473055,-0.637178482240719,
1.74218749999998));
#371121=CARTESIAN_POINT('Ctrl Pts',(1.47150067297406,-3.99080308990592E-16,
1.77968749999998));
#371122=CARTESIAN_POINT('Ctrl Pts',(1.10362550473055,0.637178482240717,
1.81718749999998));
#371123=CARTESIAN_POINT('Ctrl Pts',(0.735750336487032,1.27435696448144,
1.85468749999998));
#371124=CARTESIAN_POINT('Ctrl Pts',(0.,1.27435696448144,1.89218749999998));
#371125=CARTESIAN_POINT('Ctrl Pts',(-0.735750336487031,1.27435696448144,
1.92968749999998));
#371126=CARTESIAN_POINT('Ctrl Pts',(-1.10362550473055,0.637178482240718,
1.96718749999998));
#371127=CARTESIAN_POINT('Ctrl Pts',(-1.47150067297406,-3.84652918485864E-17,
2.00468749999998));
#371128=CARTESIAN_POINT('Ctrl Pts',(-1.10362550473055,-0.637178482240718,
2.04218749999998));
#371129=CARTESIAN_POINT('Ctrl Pts',(-0.735750336487032,-1.27435696448144,
2.07968749999998));
#371130=CARTESIAN_POINT('Ctrl Pts',(-1.56063717752333E-16,-1.27435696448144,
2.11718749999998));
#371131=CARTESIAN_POINT('Ctrl Pts',(0.735750336487031,-1.27435696448144,
2.15468749999998));
#371132=CARTESIAN_POINT('Ctrl Pts',(1.10362550473055,-0.637178482240719,
2.19218749999998));
#371133=CARTESIAN_POINT('Ctrl Pts',(1.47150067297406,-3.98677710346926E-16,
2.22968749999998));
#371134=CARTESIAN_POINT('Ctrl Pts',(1.10362550473055,0.637178482240717,
2.26718749999998));
#371135=CARTESIAN_POINT('Ctrl Pts',(0.735750336487032,1.27435696448144,
2.30468749999998));
#371136=CARTESIAN_POINT('Ctrl Pts',(0.,1.27435696448144,2.34218749999998));
#371137=CARTESIAN_POINT('Ctrl Pts',(-0.735750336487031,1.27435696448144,
2.37968749999998));
#371138=CARTESIAN_POINT('Ctrl Pts',(-1.10362550473055,0.637178482240718,
2.41718749999998));
#371139=CARTESIAN_POINT('Ctrl Pts',(-1.47150067297406,-3.80626932049204E-17,
2.45468749999998));
#371140=CARTESIAN_POINT('Ctrl Pts',(-1.10362550473055,-0.637178482240718,
2.49218749999998));
#371141=CARTESIAN_POINT('Ctrl Pts',(-0.735750336487032,-1.27435696448144,
2.52968749999998));
#371142=CARTESIAN_POINT('Ctrl Pts',(-1.56063717752333E-16,-1.27435696448144,
2.56718749999998));
#371143=CARTESIAN_POINT('Ctrl Pts',(0.735750336487031,-1.27435696448144,
2.60468749999998));
#371144=CARTESIAN_POINT('Ctrl Pts',(1.10362550473055,-0.637178482240719,
2.64218749999998));
#371145=CARTESIAN_POINT('Ctrl Pts',(1.47150067297406,-3.9827511170326E-16,
2.67968749999998));
#371146=CARTESIAN_POINT('Ctrl Pts',(1.10362550473055,0.637178482240717,
2.71718749999998));
#371147=CARTESIAN_POINT('Ctrl Pts',(0.735750336487032,1.27435696448144,
2.75468749999998));
#371148=CARTESIAN_POINT('Ctrl Pts',(0.,1.27435696448144,2.79218749999998));
#371149=CARTESIAN_POINT('Ctrl Pts',(-0.735750336487031,1.27435696448144,
2.82968749999998));
#371150=CARTESIAN_POINT('Ctrl Pts',(-1.10362550473055,0.637178482240718,
2.86718749999998));
#371151=CARTESIAN_POINT('Ctrl Pts',(-1.47150067297406,-3.76600945612543E-17,
2.90468749999998));
#371152=CARTESIAN_POINT('Ctrl Pts',(-1.10362550473055,-0.637178482240718,
2.94218749999998));
#371153=CARTESIAN_POINT('Ctrl Pts',(-0.735750336487032,-1.27435696448144,
2.97968749999998));
#371154=CARTESIAN_POINT('Ctrl Pts',(-1.56063717752333E-16,-1.27435696448144,
3.01718749999998));
#371155=CARTESIAN_POINT('Ctrl Pts',(0.735750336487031,-1.27435696448144,
3.05468749999998));
#371156=CARTESIAN_POINT('Ctrl Pts',(1.10362550473055,-0.637178482240719,
3.09218749999998));
#371157=CARTESIAN_POINT('Ctrl Pts',(1.47150067297406,-3.97872513059594E-16,
3.12968749999998));
#371158=CARTESIAN_POINT('Ctrl Pts',(1.10362550473055,0.637178482240717,
3.16718749999998));
#371159=CARTESIAN_POINT('Ctrl Pts',(0.735750336487032,1.27435696448144,
3.20468749999998));
#371160=CARTESIAN_POINT('Ctrl Pts',(0.,1.27435696448144,3.24218749999998));
#371161=CARTESIAN_POINT('Ctrl Pts',(-0.735750336487031,1.27435696448144,
3.27968749999998));
#371162=CARTESIAN_POINT('Ctrl Pts',(-1.10362550473055,0.637178482240718,
3.31718749999998));
#371163=CARTESIAN_POINT('Ctrl Pts',(-1.47150067297406,-3.72574959175883E-17,
3.35468749999998));
#371164=CARTESIAN_POINT('Ctrl Pts',(-1.10362550473055,-0.637178482240718,
3.39218749999998));
#371165=CARTESIAN_POINT('Ctrl Pts',(-0.735750336487032,-1.27435696448144,
3.42968749999998));
#371166=CARTESIAN_POINT('Ctrl Pts',(-1.56063717752333E-16,-1.27435696448144,
3.46718749999998));
#371167=CARTESIAN_POINT('Ctrl Pts',(0.735750336487031,-1.27435696448144,
3.50468749999998));
#371168=CARTESIAN_POINT('Ctrl Pts',(1.10362550473055,-0.637178482240719,
3.54218749999998));
#371169=CARTESIAN_POINT('Ctrl Pts',(1.33552814991602,-0.235511318369856,
3.56582690256139));
#371170=CARTESIAN_POINT('Ctrl Pts',(1.25500358340531,0.221250262287215,
3.59270878848825));
#371171=CARTESIAN_POINT('Ctrl Pts',(1.12949581523918,0.933171220777297,
3.6346076232535));
#371172=CARTESIAN_POINT('Ctrl Pts',(1.00398804707305,1.64509217926738,3.67650645801875));
#371173=CARTESIAN_POINT('Origin',(1.38777878078145E-16,1.38777878078145E-16,
-4.19687500000002));
#371174=CARTESIAN_POINT('Ctrl Pts',(-0.155365792422873,-0.945030276552907,
-3.95478357377727));
#371175=CARTESIAN_POINT('Ctrl Pts',(-0.0782008300208539,-0.957716426222737,
-3.94905354577365));
#371176=CARTESIAN_POINT('Ctrl Pts',(-1.17286435586452E-16,-0.957716426222737,
-3.94375000000002));
#371177=CARTESIAN_POINT('Ctrl Pts',(0.,1.27435696448144,-3.98593750000002));
#371178=CARTESIAN_POINT('Ctrl Pts',(-0.735750336487031,1.27435696448144,
-3.94843750000002));
#371179=CARTESIAN_POINT('Ctrl Pts',(-1.10362550473055,0.637178482240718,
-3.91093750000002));
#371180=CARTESIAN_POINT('Ctrl Pts',(-1.47150067297406,-4.37242366314742E-17,
-3.87343750000002));
#371181=CARTESIAN_POINT('Ctrl Pts',(-1.10362550473055,-0.637178482240718,
-3.83593750000002));
#371182=CARTESIAN_POINT('Ctrl Pts',(-0.735750336487032,-1.27435696448144,
-3.79843750000002));
#371183=CARTESIAN_POINT('Ctrl Pts',(-1.56063717752333E-16,-1.27435696448144,
-3.76093750000002));
#371184=CARTESIAN_POINT('Ctrl Pts',(0.735750336487031,-1.27435696448144,
-3.72343750000002));
#371185=CARTESIAN_POINT('Ctrl Pts',(1.10362550473055,-0.637178482240719,
-3.68593750000002));
#371186=CARTESIAN_POINT('Ctrl Pts',(1.47150067297406,-4.03936655129813E-16,
-3.64843750000002));
#371187=CARTESIAN_POINT('Ctrl Pts',(1.10362550473055,0.637178482240717,
-3.61093750000002));
#371188=CARTESIAN_POINT('Ctrl Pts',(0.735750336487032,1.27435696448144,
-3.57343750000002));
#371189=CARTESIAN_POINT('Ctrl Pts',(0.,1.27435696448144,-3.53593750000002));
#371190=CARTESIAN_POINT('Ctrl Pts',(-0.735750336487031,1.27435696448144,
-3.49843750000002));
#371191=CARTESIAN_POINT('Ctrl Pts',(-1.10362550473055,0.637178482240718,
-3.46093750000002));
#371192=CARTESIAN_POINT('Ctrl Pts',(-1.47150067297406,-4.33216379878081E-17,
-3.42343750000002));
#371193=CARTESIAN_POINT('Ctrl Pts',(-1.10362550473055,-0.637178482240718,
-3.38593750000002));
#371194=CARTESIAN_POINT('Ctrl Pts',(-0.735750336487032,-1.27435696448144,
-3.34843750000002));
#371195=CARTESIAN_POINT('Ctrl Pts',(-1.56063717752333E-16,-1.27435696448144,
-3.31093750000002));
#371196=CARTESIAN_POINT('Ctrl Pts',(0.735750336487031,-1.27435696448144,
-3.27343750000002));
#371197=CARTESIAN_POINT('Ctrl Pts',(1.10362550473055,-0.637178482240719,
-3.23593750000002));
#371198=CARTESIAN_POINT('Ctrl Pts',(1.47150067297406,-4.03534056486148E-16,
-3.19843750000002));
#371199=CARTESIAN_POINT('Ctrl Pts',(1.10362550473055,0.637178482240717,
-3.16093750000002));
#371200=CARTESIAN_POINT('Ctrl Pts',(0.735750336487032,1.27435696448144,
-3.12343750000002));
#371201=CARTESIAN_POINT('Ctrl Pts',(0.,1.27435696448144,-3.08593750000002));
#371202=CARTESIAN_POINT('Ctrl Pts',(-0.735750336487031,1.27435696448144,
-3.04843750000002));
#371203=CARTESIAN_POINT('Ctrl Pts',(-1.10362550473055,0.637178482240718,
-3.01093750000002));
#371204=CARTESIAN_POINT('Ctrl Pts',(-1.47150067297406,-4.29190393441421E-17,
-2.97343750000002));
#371205=CARTESIAN_POINT('Ctrl Pts',(-1.10362550473055,-0.637178482240718,
-2.93593750000002));
#371206=CARTESIAN_POINT('Ctrl Pts',(-0.735750336487032,-1.27435696448144,
-2.89843750000002));
#371207=CARTESIAN_POINT('Ctrl Pts',(-1.56063717752333E-16,-1.27435696448144,
-2.86093750000002));
#371208=CARTESIAN_POINT('Ctrl Pts',(0.735750336487031,-1.27435696448144,
-2.82343750000002));
#371209=CARTESIAN_POINT('Ctrl Pts',(1.10362550473055,-0.637178482240719,
-2.78593750000002));
#371210=CARTESIAN_POINT('Ctrl Pts',(1.47150067297406,-4.03131457842481E-16,
-2.74843750000002));
#371211=CARTESIAN_POINT('Ctrl Pts',(1.10362550473055,0.637178482240717,
-2.71093750000002));
#371212=CARTESIAN_POINT('Ctrl Pts',(0.735750336487032,1.27435696448144,
-2.67343750000002));
#371213=CARTESIAN_POINT('Ctrl Pts',(0.,1.27435696448144,-2.63593750000002));
#371214=CARTESIAN_POINT('Ctrl Pts',(-0.735750336487031,1.27435696448144,
-2.59843750000002));
#371215=CARTESIAN_POINT('Ctrl Pts',(-1.10362550473055,0.637178482240718,
-2.56093750000002));
#371216=CARTESIAN_POINT('Ctrl Pts',(-1.47150067297406,-4.2516440700476E-17,
-2.52343750000002));
#371217=CARTESIAN_POINT('Ctrl Pts',(-1.10362550473055,-0.637178482240718,
-2.48593750000002));
#371218=CARTESIAN_POINT('Ctrl Pts',(-0.735750336487032,-1.27435696448144,
-2.44843750000002));
#371219=CARTESIAN_POINT('Ctrl Pts',(-1.56063717752333E-16,-1.27435696448144,
-2.41093750000002));
#371220=CARTESIAN_POINT('Ctrl Pts',(0.735750336487031,-1.27435696448144,
-2.37343750000002));
#371221=CARTESIAN_POINT('Ctrl Pts',(1.10362550473055,-0.637178482240719,
-2.33593750000002));
#371222=CARTESIAN_POINT('Ctrl Pts',(1.47150067297406,-4.02728859198815E-16,
-2.29843750000002));
#371223=CARTESIAN_POINT('Ctrl Pts',(1.10362550473055,0.637178482240717,
-2.26093750000002));
#371224=CARTESIAN_POINT('Ctrl Pts',(0.735750336487032,1.27435696448144,
-2.22343750000002));
#371225=CARTESIAN_POINT('Ctrl Pts',(0.,1.27435696448144,-2.18593750000002));
#371226=CARTESIAN_POINT('Ctrl Pts',(-0.735750336487031,1.27435696448144,
-2.14843750000002));
#371227=CARTESIAN_POINT('Ctrl Pts',(-1.10362550473055,0.637178482240718,
-2.11093750000002));
#371228=CARTESIAN_POINT('Ctrl Pts',(-1.47150067297406,-4.211384205681E-17,
-2.07343750000002));
#371229=CARTESIAN_POINT('Ctrl Pts',(-1.10362550473055,-0.637178482240718,
-2.03593750000002));
#371230=CARTESIAN_POINT('Ctrl Pts',(-0.735750336487032,-1.27435696448144,
-1.99843750000002));
#371231=CARTESIAN_POINT('Ctrl Pts',(-1.56063717752333E-16,-1.27435696448144,
-1.96093750000002));
#371232=CARTESIAN_POINT('Ctrl Pts',(0.735750336487031,-1.27435696448144,
-1.92343750000002));
#371233=CARTESIAN_POINT('Ctrl Pts',(1.10362550473055,-0.637178482240719,
-1.88593750000002));
#371234=CARTESIAN_POINT('Ctrl Pts',(1.47150067297406,-4.02326260555149E-16,
-1.84843750000002));
#371235=CARTESIAN_POINT('Ctrl Pts',(1.10362550473055,0.637178482240717,
-1.81093750000002));
#371236=CARTESIAN_POINT('Ctrl Pts',(0.735750336487032,1.27435696448144,
-1.77343750000002));
#371237=CARTESIAN_POINT('Ctrl Pts',(0.,1.27435696448144,-1.73593750000002));
#371238=CARTESIAN_POINT('Ctrl Pts',(-0.735750336487031,1.27435696448144,
-1.69843750000002));
#371239=CARTESIAN_POINT('Ctrl Pts',(-1.10362550473055,0.637178482240718,
-1.66093750000002));
#371240=CARTESIAN_POINT('Ctrl Pts',(-1.47150067297406,-4.17112434131439E-17,
-1.62343750000002));
#371241=CARTESIAN_POINT('Ctrl Pts',(-1.10362550473055,-0.637178482240718,
-1.58593750000002));
#371242=CARTESIAN_POINT('Ctrl Pts',(-0.735750336487032,-1.27435696448144,
-1.54843750000002));
#371243=CARTESIAN_POINT('Ctrl Pts',(-1.56063717752333E-16,-1.27435696448144,
-1.51093750000002));
#371244=CARTESIAN_POINT('Ctrl Pts',(0.735750336487031,-1.27435696448144,
-1.47343750000002));
#371245=CARTESIAN_POINT('Ctrl Pts',(1.10362550473055,-0.637178482240719,
-1.43593750000002));
#371246=CARTESIAN_POINT('Ctrl Pts',(1.47150067297406,-4.01923661911483E-16,
-1.39843750000002));
#371247=CARTESIAN_POINT('Ctrl Pts',(1.10362550473055,0.637178482240717,
-1.36093750000002));
#371248=CARTESIAN_POINT('Ctrl Pts',(0.735750336487032,1.27435696448144,
-1.32343750000002));
#371249=CARTESIAN_POINT('Ctrl Pts',(0.,1.27435696448144,-1.28593750000002));
#371250=CARTESIAN_POINT('Ctrl Pts',(-0.735750336487031,1.27435696448144,
-1.24843750000002));
#371251=CARTESIAN_POINT('Ctrl Pts',(-1.10362550473055,0.637178482240718,
-1.21093750000002));
#371252=CARTESIAN_POINT('Ctrl Pts',(-1.47150067297406,-4.13086447694779E-17,
-1.17343750000002));
#371253=CARTESIAN_POINT('Ctrl Pts',(-1.10362550473055,-0.637178482240718,
-1.13593750000002));
#371254=CARTESIAN_POINT('Ctrl Pts',(-0.735750336487032,-1.27435696448144,
-1.09843750000002));
#371255=CARTESIAN_POINT('Ctrl Pts',(-1.56063717752333E-16,-1.27435696448144,
-1.06093750000002));
#371256=CARTESIAN_POINT('Ctrl Pts',(0.735750336487031,-1.27435696448144,
-1.02343750000002));
#371257=CARTESIAN_POINT('Ctrl Pts',(1.10362550473055,-0.637178482240719,
-0.985937500000016));
#371258=CARTESIAN_POINT('Ctrl Pts',(1.47150067297406,-4.01521063267817E-16,
-0.948437500000016));
#371259=CARTESIAN_POINT('Ctrl Pts',(1.10362550473055,0.637178482240717,
-0.910937500000016));
#371260=CARTESIAN_POINT('Ctrl Pts',(0.735750336487032,1.27435696448144,
-0.873437500000016));
#371261=CARTESIAN_POINT('Ctrl Pts',(0.,1.27435696448144,-0.835937500000016));
#371262=CARTESIAN_POINT('Ctrl Pts',(-0.735750336487031,1.27435696448144,
-0.798437500000016));
#371263=CARTESIAN_POINT('Ctrl Pts',(-1.10362550473055,0.637178482240718,
-0.760937500000016));
#371264=CARTESIAN_POINT('Ctrl Pts',(-1.47150067297406,-4.09060461258118E-17,
-0.723437500000016));
#371265=CARTESIAN_POINT('Ctrl Pts',(-1.10362550473055,-0.637178482240718,
-0.685937500000016));
#371266=CARTESIAN_POINT('Ctrl Pts',(-0.735750336487032,-1.27435696448144,
-0.648437500000016));
#371267=CARTESIAN_POINT('Ctrl Pts',(-1.56063717752333E-16,-1.27435696448144,
-0.610937500000016));
#371268=CARTESIAN_POINT('Ctrl Pts',(0.735750336487031,-1.27435696448144,
-0.573437500000016));
#371269=CARTESIAN_POINT('Ctrl Pts',(1.10362550473055,-0.637178482240719,
-0.535937500000016));
#371270=CARTESIAN_POINT('Ctrl Pts',(1.47150067297406,-4.01118464624151E-16,
-0.498437500000016));
#371271=CARTESIAN_POINT('Ctrl Pts',(1.10362550473055,0.637178482240717,
-0.460937500000016));
#371272=CARTESIAN_POINT('Ctrl Pts',(0.735750336487032,1.27435696448144,
-0.423437500000016));
#371273=CARTESIAN_POINT('Ctrl Pts',(0.,1.27435696448144,-0.385937500000016));
#371274=CARTESIAN_POINT('Ctrl Pts',(-0.735750336487031,1.27435696448144,
-0.348437500000016));
#371275=CARTESIAN_POINT('Ctrl Pts',(-1.10362550473055,0.637178482240718,
-0.310937500000016));
#371276=CARTESIAN_POINT('Ctrl Pts',(-1.47150067297406,-4.05034474821458E-17,
-0.273437500000016));
#371277=CARTESIAN_POINT('Ctrl Pts',(-1.10362550473055,-0.637178482240718,
-0.235937500000016));
#371278=CARTESIAN_POINT('Ctrl Pts',(-0.735750336487032,-1.27435696448144,
-0.198437500000016));
#371279=CARTESIAN_POINT('Ctrl Pts',(-1.56063717752333E-16,-1.27435696448144,
-0.160937500000016));
#371280=CARTESIAN_POINT('Ctrl Pts',(0.735750336487031,-1.27435696448144,
-0.123437500000016));
#371281=CARTESIAN_POINT('Ctrl Pts',(1.10362550473055,-0.637178482240719,
-0.0859375000000157));
#371282=CARTESIAN_POINT('Ctrl Pts',(1.47150067297406,-4.00715865980485E-16,
-0.0484375000000155));
#371283=CARTESIAN_POINT('Ctrl Pts',(1.10362550473055,0.637178482240717,
-0.0109375000000161));
#371284=CARTESIAN_POINT('Ctrl Pts',(0.735750336487032,1.27435696448144,
0.0265624999999841));
#371285=CARTESIAN_POINT('Ctrl Pts',(0.,1.27435696448144,0.0640624999999843));
#371286=CARTESIAN_POINT('Ctrl Pts',(-0.735750336487031,1.27435696448144,
0.101562499999984));
#371287=CARTESIAN_POINT('Ctrl Pts',(-1.10362550473055,0.637178482240718,
0.139062499999984));
#371288=CARTESIAN_POINT('Ctrl Pts',(-1.47150067297406,-4.01008488384797E-17,
0.176562499999984));
#371289=CARTESIAN_POINT('Ctrl Pts',(-1.10362550473055,-0.637178482240718,
0.214062499999984));
#371290=CARTESIAN_POINT('Ctrl Pts',(-0.735750336487032,-1.27435696448144,
0.251562499999984));
#371291=CARTESIAN_POINT('Ctrl Pts',(-1.56063717752333E-16,-1.27435696448144,
0.289062499999984));
#371292=CARTESIAN_POINT('Ctrl Pts',(0.735750336487031,-1.27435696448144,
0.326562499999984));
#371293=CARTESIAN_POINT('Ctrl Pts',(1.10362550473055,-0.637178482240719,
0.364062499999984));
#371294=CARTESIAN_POINT('Ctrl Pts',(1.47150067297406,-4.00313267336819E-16,
0.401562499999984));
#371295=CARTESIAN_POINT('Ctrl Pts',(1.10362550473055,0.637178482240717,
0.439062499999984));
#371296=CARTESIAN_POINT('Ctrl Pts',(0.735750336487032,1.27435696448144,
0.476562499999984));
#371297=CARTESIAN_POINT('Ctrl Pts',(0.,1.27435696448144,0.514062499999984));
#371298=CARTESIAN_POINT('Ctrl Pts',(-0.735750336487031,1.27435696448144,
0.551562499999984));
#371299=CARTESIAN_POINT('Ctrl Pts',(-1.10362550473055,0.637178482240718,
0.589062499999984));
#371300=CARTESIAN_POINT('Ctrl Pts',(-1.47150067297406,-3.96982501948137E-17,
0.626562499999984));
#371301=CARTESIAN_POINT('Ctrl Pts',(-1.10362550473055,-0.637178482240718,
0.664062499999984));
#371302=CARTESIAN_POINT('Ctrl Pts',(-0.735750336487032,-1.27435696448144,
0.701562499999984));
#371303=CARTESIAN_POINT('Ctrl Pts',(-1.56063717752333E-16,-1.27435696448144,
0.739062499999984));
#371304=CARTESIAN_POINT('Ctrl Pts',(0.735750336487031,-1.27435696448144,
0.776562499999984));
#371305=CARTESIAN_POINT('Ctrl Pts',(1.10362550473055,-0.637178482240719,
0.814062499999984));
#371306=CARTESIAN_POINT('Ctrl Pts',(1.47150067297406,-3.99910668693153E-16,
0.851562499999984));
#371307=CARTESIAN_POINT('Ctrl Pts',(1.10362550473055,0.637178482240717,
0.889062499999985));
#371308=CARTESIAN_POINT('Ctrl Pts',(0.735750336487032,1.27435696448144,
0.926562499999984));
#371309=CARTESIAN_POINT('Ctrl Pts',(0.,1.27435696448144,0.964062499999984));
#371310=CARTESIAN_POINT('Ctrl Pts',(-0.735750336487031,1.27435696448144,
1.00156249999998));
#371311=CARTESIAN_POINT('Ctrl Pts',(-1.10362550473055,0.637178482240718,
1.03906249999998));
#371312=CARTESIAN_POINT('Ctrl Pts',(-1.47150067297406,-3.92956515511476E-17,
1.07656249999998));
#371313=CARTESIAN_POINT('Ctrl Pts',(-1.10362550473055,-0.637178482240718,
1.11406249999998));
#371314=CARTESIAN_POINT('Ctrl Pts',(-0.735750336487032,-1.27435696448144,
1.15156249999998));
#371315=CARTESIAN_POINT('Ctrl Pts',(-1.56063717752333E-16,-1.27435696448144,
1.18906249999998));
#371316=CARTESIAN_POINT('Ctrl Pts',(0.735750336487031,-1.27435696448144,
1.22656249999998));
#371317=CARTESIAN_POINT('Ctrl Pts',(1.10362550473055,-0.637178482240719,
1.26406249999998));
#371318=CARTESIAN_POINT('Ctrl Pts',(1.47150067297406,-3.99508070049487E-16,
1.30156249999998));
#371319=CARTESIAN_POINT('Ctrl Pts',(1.10362550473055,0.637178482240717,
1.33906249999998));
#371320=CARTESIAN_POINT('Ctrl Pts',(0.735750336487032,1.27435696448144,
1.37656249999998));
#371321=CARTESIAN_POINT('Ctrl Pts',(0.,1.27435696448144,1.41406249999998));
#371322=CARTESIAN_POINT('Ctrl Pts',(-0.735750336487031,1.27435696448144,
1.45156249999998));
#371323=CARTESIAN_POINT('Ctrl Pts',(-1.10362550473055,0.637178482240718,
1.48906249999998));
#371324=CARTESIAN_POINT('Ctrl Pts',(-1.47150067297406,-3.88930529074816E-17,
1.52656249999998));
#371325=CARTESIAN_POINT('Ctrl Pts',(-1.10362550473055,-0.637178482240718,
1.56406249999998));
#371326=CARTESIAN_POINT('Ctrl Pts',(-0.735750336487032,-1.27435696448144,
1.60156249999998));
#371327=CARTESIAN_POINT('Ctrl Pts',(-1.56063717752333E-16,-1.27435696448144,
1.63906249999998));
#371328=CARTESIAN_POINT('Ctrl Pts',(0.735750336487031,-1.27435696448144,
1.67656249999998));
#371329=CARTESIAN_POINT('Ctrl Pts',(1.10362550473055,-0.637178482240719,
1.71406249999998));
#371330=CARTESIAN_POINT('Ctrl Pts',(1.47150067297406,-3.99105471405821E-16,
1.75156249999998));
#371331=CARTESIAN_POINT('Ctrl Pts',(1.10362550473055,0.637178482240717,
1.78906249999998));
#371332=CARTESIAN_POINT('Ctrl Pts',(0.735750336487032,1.27435696448144,
1.82656249999998));
#371333=CARTESIAN_POINT('Ctrl Pts',(0.,1.27435696448144,1.86406249999998));
#371334=CARTESIAN_POINT('Ctrl Pts',(-0.735750336487031,1.27435696448144,
1.90156249999998));
#371335=CARTESIAN_POINT('Ctrl Pts',(-1.10362550473055,0.637178482240718,
1.93906249999998));
#371336=CARTESIAN_POINT('Ctrl Pts',(-1.47150067297406,-3.84904542638155E-17,
1.97656249999998));
#371337=CARTESIAN_POINT('Ctrl Pts',(-1.10362550473055,-0.637178482240718,
2.01406249999998));
#371338=CARTESIAN_POINT('Ctrl Pts',(-0.735750336487032,-1.27435696448144,
2.05156249999998));
#371339=CARTESIAN_POINT('Ctrl Pts',(-1.56063717752333E-16,-1.27435696448144,
2.08906249999998));
#371340=CARTESIAN_POINT('Ctrl Pts',(0.735750336487031,-1.27435696448144,
2.12656249999998));
#371341=CARTESIAN_POINT('Ctrl Pts',(1.10362550473055,-0.637178482240719,
2.16406249999998));
#371342=CARTESIAN_POINT('Ctrl Pts',(1.47150067297406,-3.98702872762155E-16,
2.20156249999998));
#371343=CARTESIAN_POINT('Ctrl Pts',(1.10362550473055,0.637178482240717,
2.23906249999998));
#371344=CARTESIAN_POINT('Ctrl Pts',(0.735750336487032,1.27435696448144,
2.27656249999998));
#371345=CARTESIAN_POINT('Ctrl Pts',(0.,1.27435696448144,2.31406249999998));
#371346=CARTESIAN_POINT('Ctrl Pts',(-0.735750336487031,1.27435696448144,
2.35156249999998));
#371347=CARTESIAN_POINT('Ctrl Pts',(-1.10362550473055,0.637178482240718,
2.38906249999998));
#371348=CARTESIAN_POINT('Ctrl Pts',(-1.47150067297406,-3.80878556201495E-17,
2.42656249999998));
#371349=CARTESIAN_POINT('Ctrl Pts',(-1.10362550473055,-0.637178482240718,
2.46406249999998));
#371350=CARTESIAN_POINT('Ctrl Pts',(-0.735750336487032,-1.27435696448144,
2.50156249999998));
#371351=CARTESIAN_POINT('Ctrl Pts',(-1.56063717752333E-16,-1.27435696448144,
2.53906249999998));
#371352=CARTESIAN_POINT('Ctrl Pts',(0.735750336487031,-1.27435696448144,
2.57656249999998));
#371353=CARTESIAN_POINT('Ctrl Pts',(1.10362550473055,-0.637178482240719,
2.61406249999998));
#371354=CARTESIAN_POINT('Ctrl Pts',(1.47150067297406,-3.98300274118489E-16,
2.65156249999998));
#371355=CARTESIAN_POINT('Ctrl Pts',(1.10362550473055,0.637178482240717,
2.68906249999998));
#371356=CARTESIAN_POINT('Ctrl Pts',(0.735750336487032,1.27435696448144,
2.72656249999998));
#371357=CARTESIAN_POINT('Ctrl Pts',(0.,1.27435696448144,2.76406249999998));
#371358=CARTESIAN_POINT('Ctrl Pts',(-0.735750336487031,1.27435696448144,
2.80156249999998));
#371359=CARTESIAN_POINT('Ctrl Pts',(-1.10362550473055,0.637178482240718,
2.83906249999998));
#371360=CARTESIAN_POINT('Ctrl Pts',(-1.47150067297406,-3.76852569764834E-17,
2.87656249999998));
#371361=CARTESIAN_POINT('Ctrl Pts',(-1.10362550473055,-0.637178482240718,
2.91406249999998));
#371362=CARTESIAN_POINT('Ctrl Pts',(-0.735750336487032,-1.27435696448144,
2.95156249999998));
#371363=CARTESIAN_POINT('Ctrl Pts',(-1.56063717752333E-16,-1.27435696448144,
2.98906249999998));
#371364=CARTESIAN_POINT('Ctrl Pts',(0.735750336487031,-1.27435696448144,
3.02656249999998));
#371365=CARTESIAN_POINT('Ctrl Pts',(1.10362550473055,-0.637178482240719,
3.06406249999998));
#371366=CARTESIAN_POINT('Ctrl Pts',(1.47150067297406,-3.97897675474823E-16,
3.10156249999998));
#371367=CARTESIAN_POINT('Ctrl Pts',(1.10362550473055,0.637178482240717,
3.13906249999998));
#371368=CARTESIAN_POINT('Ctrl Pts',(0.735750336487032,1.27435696448144,
3.17656249999998));
#371369=CARTESIAN_POINT('Ctrl Pts',(0.,1.27435696448144,3.21406249999998));
#371370=CARTESIAN_POINT('Ctrl Pts',(-0.735750336487031,1.27435696448144,
3.25156249999998));
#371371=CARTESIAN_POINT('Ctrl Pts',(-1.10362550473055,0.637178482240718,
3.28906249999998));
#371372=CARTESIAN_POINT('Ctrl Pts',(-1.47150067297406,-3.72826583328174E-17,
3.32656249999998));
#371373=CARTESIAN_POINT('Ctrl Pts',(-1.10362550473055,-0.637178482240718,
3.36406249999998));
#371374=CARTESIAN_POINT('Ctrl Pts',(-0.735750336487032,-1.27435696448144,
3.40156249999998));
#371375=CARTESIAN_POINT('Ctrl Pts',(-1.56063717752333E-16,-1.27435696448144,
3.43906249999998));
#371376=CARTESIAN_POINT('Ctrl Pts',(0.735750336487031,-1.27435696448144,
3.47656249999998));
#371377=CARTESIAN_POINT('Ctrl Pts',(1.10362550473055,-0.637178482240719,
3.51406249999998));
#371378=CARTESIAN_POINT('Ctrl Pts',(1.47150067297406,-3.97495076831157E-16,
3.55156249999998));
#371379=CARTESIAN_POINT('Ctrl Pts',(1.10362550473055,0.637178482240717,
3.58906249999998));
#371380=CARTESIAN_POINT('Ctrl Pts',(0.735750336487032,1.27435696448144,
3.62656249999998));
#371381=CARTESIAN_POINT('Ctrl Pts',(0.,1.27435696448144,3.66406249999998));
#371382=CARTESIAN_POINT('Ctrl Pts',(-0.735750336487031,1.27435696448144,
3.70156249999998));
#371383=CARTESIAN_POINT('Ctrl Pts',(-1.10362550473055,0.637178482240718,
3.73906249999998));
#371384=CARTESIAN_POINT('Ctrl Pts',(-1.47150067297406,-3.68800596891513E-17,
3.77656249999998));
#371385=CARTESIAN_POINT('Ctrl Pts',(-1.10362550473055,-0.637178482240718,
3.81406249999998));
#371386=CARTESIAN_POINT('Ctrl Pts',(-0.735750336487032,-1.27435696448144,
3.85156249999998));
#371387=CARTESIAN_POINT('Ctrl Pts',(-1.56063717752333E-16,-1.27435696448144,
3.88906249999998));
#371388=CARTESIAN_POINT('Ctrl Pts',(0.735750336487031,-1.27435696448144,
3.92656249999998));
#371389=CARTESIAN_POINT('Ctrl Pts',(1.10362550473055,-0.637178482240719,
3.96406249999998));
#371390=CARTESIAN_POINT('Ctrl Pts',(1.33553307714466,-0.235502784159521,
3.98770240482708));
#371391=CARTESIAN_POINT('Ctrl Pts',(1.2550005617303,0.22126740152805,4.01458479718761));
#371392=CARTESIAN_POINT('Ctrl Pts',(0.,0.957716426222737,-4.16875000000002));
#371393=CARTESIAN_POINT('Ctrl Pts',(-0.552937836487023,0.957716426222737,
-4.13125000000002));
#371394=CARTESIAN_POINT('Ctrl Pts',(-0.829406754730535,0.478858213111368,
-4.09375000000002));
#371395=CARTESIAN_POINT('Ctrl Pts',(-1.10587567297405,-6.6275866627377E-17,
-4.05625000000002));
#371396=CARTESIAN_POINT('Ctrl Pts',(-0.829406754730535,-0.478858213111368,
-4.01875000000002));
#371397=CARTESIAN_POINT('Ctrl Pts',(-0.552937836487024,-0.957716426222737,
-3.98125000000002));
#371398=CARTESIAN_POINT('Ctrl Pts',(-1.17286435586452E-16,-0.957716426222737,
-3.94375000000002));
#371399=CARTESIAN_POINT('Ctrl Pts',(0.552937836487023,-0.957716426222737,
-3.90625000000002));
#371400=CARTESIAN_POINT('Ctrl Pts',(0.829406754730535,-0.478858213111369,
-3.86875000000002));
#371401=CARTESIAN_POINT('Ctrl Pts',(1.10587567297405,-3.36935987938062E-16,
-3.83125000000002));
#371402=CARTESIAN_POINT('Ctrl Pts',(0.829406754730536,0.478858213111368,
-3.79375000000002));
#371403=CARTESIAN_POINT('Ctrl Pts',(0.552937836487024,0.957716426222737,
-3.75625000000002));
#371404=CARTESIAN_POINT('Ctrl Pts',(0.,0.957716426222737,-3.71875000000002));
#371405=CARTESIAN_POINT('Ctrl Pts',(-0.552937836487023,0.957716426222737,
-3.68125000000002));
#371406=CARTESIAN_POINT('Ctrl Pts',(-0.829406754730535,0.478858213111368,
-3.64375000000002));
#371407=CARTESIAN_POINT('Ctrl Pts',(-1.10587567297405,-6.5873267983711E-17,
-3.60625000000002));
#371408=CARTESIAN_POINT('Ctrl Pts',(-0.829406754730535,-0.478858213111368,
-3.56875000000002));
#371409=CARTESIAN_POINT('Ctrl Pts',(-0.552937836487024,-0.957716426222737,
-3.53125000000002));
#371410=CARTESIAN_POINT('Ctrl Pts',(-1.17286435586452E-16,-0.957716426222737,
-3.49375000000002));
#371411=CARTESIAN_POINT('Ctrl Pts',(0.552937836487023,-0.957716426222737,
-3.45625000000002));
#371412=CARTESIAN_POINT('Ctrl Pts',(0.829406754730535,-0.478858213111369,
-3.41875000000002));
#371413=CARTESIAN_POINT('Ctrl Pts',(1.10587567297405,-3.36533389294396E-16,
-3.38125000000002));
#371414=CARTESIAN_POINT('Ctrl Pts',(0.829406754730536,0.478858213111368,
-3.34375000000002));
#371415=CARTESIAN_POINT('Ctrl Pts',(0.552937836487024,0.957716426222737,
-3.30625000000002));
#371416=CARTESIAN_POINT('Ctrl Pts',(0.,0.957716426222737,-3.26875000000002));
#371417=CARTESIAN_POINT('Ctrl Pts',(-0.552937836487023,0.957716426222737,
-3.23125000000002));
#371418=CARTESIAN_POINT('Ctrl Pts',(-0.829406754730535,0.478858213111368,
-3.19375000000002));
#371419=CARTESIAN_POINT('Ctrl Pts',(-1.10587567297405,-6.54706693400449E-17,
-3.15625000000002));
#371420=CARTESIAN_POINT('Ctrl Pts',(-0.829406754730535,-0.478858213111368,
-3.11875000000002));
#371421=CARTESIAN_POINT('Ctrl Pts',(-0.552937836487024,-0.957716426222737,
-3.08125000000002));
#371422=CARTESIAN_POINT('Ctrl Pts',(-1.17286435586452E-16,-0.957716426222737,
-3.04375000000002));
#371423=CARTESIAN_POINT('Ctrl Pts',(0.552937836487023,-0.957716426222737,
-3.00625000000002));
#371424=CARTESIAN_POINT('Ctrl Pts',(0.829406754730535,-0.478858213111369,
-2.96875000000002));
#371425=CARTESIAN_POINT('Ctrl Pts',(1.10587567297405,-3.3613079065073E-16,
-2.93125000000002));
#371426=CARTESIAN_POINT('Ctrl Pts',(0.829406754730536,0.478858213111368,
-2.89375000000002));
#371427=CARTESIAN_POINT('Ctrl Pts',(0.552937836487024,0.957716426222737,
-2.85625000000002));
#371428=CARTESIAN_POINT('Ctrl Pts',(0.,0.957716426222737,-2.81875000000002));
#371429=CARTESIAN_POINT('Ctrl Pts',(-0.552937836487023,0.957716426222737,
-2.78125000000002));
#371430=CARTESIAN_POINT('Ctrl Pts',(-0.829406754730535,0.478858213111368,
-2.74375000000002));
#371431=CARTESIAN_POINT('Ctrl Pts',(-1.10587567297405,-6.50680706963789E-17,
-2.70625000000002));
#371432=CARTESIAN_POINT('Ctrl Pts',(-0.829406754730535,-0.478858213111368,
-2.66875000000002));
#371433=CARTESIAN_POINT('Ctrl Pts',(-0.552937836487024,-0.957716426222737,
-2.63125000000002));
#371434=CARTESIAN_POINT('Ctrl Pts',(-1.17286435586452E-16,-0.957716426222737,
-2.59375000000002));
#371435=CARTESIAN_POINT('Ctrl Pts',(0.552937836487023,-0.957716426222737,
-2.55625000000002));
#371436=CARTESIAN_POINT('Ctrl Pts',(0.829406754730535,-0.478858213111369,
-2.51875000000002));
#371437=CARTESIAN_POINT('Ctrl Pts',(1.10587567297405,-3.35728192007064E-16,
-2.48125000000002));
#371438=CARTESIAN_POINT('Ctrl Pts',(0.829406754730536,0.478858213111368,
-2.44375000000002));
#371439=CARTESIAN_POINT('Ctrl Pts',(0.552937836487024,0.957716426222737,
-2.40625000000002));
#371440=CARTESIAN_POINT('Ctrl Pts',(0.,0.957716426222737,-2.36875000000002));
#371441=CARTESIAN_POINT('Ctrl Pts',(-0.552937836487023,0.957716426222737,
-2.33125000000002));
#371442=CARTESIAN_POINT('Ctrl Pts',(-0.829406754730535,0.478858213111368,
-2.29375000000002));
#371443=CARTESIAN_POINT('Ctrl Pts',(-1.10587567297405,-6.46654720527128E-17,
-2.25625000000002));
#371444=CARTESIAN_POINT('Ctrl Pts',(-0.829406754730535,-0.478858213111368,
-2.21875000000002));
#371445=CARTESIAN_POINT('Ctrl Pts',(-0.552937836487024,-0.957716426222737,
-2.18125000000002));
#371446=CARTESIAN_POINT('Ctrl Pts',(-1.17286435586452E-16,-0.957716426222737,
-2.14375000000002));
#371447=CARTESIAN_POINT('Ctrl Pts',(0.552937836487023,-0.957716426222737,
-2.10625000000002));
#371448=CARTESIAN_POINT('Ctrl Pts',(0.829406754730535,-0.478858213111369,
-2.06875000000002));
#371449=CARTESIAN_POINT('Ctrl Pts',(1.10587567297405,-3.35325593363398E-16,
-2.03125000000002));
#371450=CARTESIAN_POINT('Ctrl Pts',(0.829406754730536,0.478858213111368,
-1.99375000000002));
#371451=CARTESIAN_POINT('Ctrl Pts',(0.552937836487024,0.957716426222737,
-1.95625000000002));
#371452=CARTESIAN_POINT('Ctrl Pts',(0.,0.957716426222737,-1.91875000000002));
#371453=CARTESIAN_POINT('Ctrl Pts',(-0.552937836487023,0.957716426222737,
-1.88125000000002));
#371454=CARTESIAN_POINT('Ctrl Pts',(-0.829406754730535,0.478858213111368,
-1.84375000000002));
#371455=CARTESIAN_POINT('Ctrl Pts',(-1.10587567297405,-6.42628734090468E-17,
-1.80625000000002));
#371456=CARTESIAN_POINT('Ctrl Pts',(-0.829406754730535,-0.478858213111368,
-1.76875000000002));
#371457=CARTESIAN_POINT('Ctrl Pts',(-0.552937836487024,-0.957716426222737,
-1.73125000000002));
#371458=CARTESIAN_POINT('Ctrl Pts',(-1.17286435586452E-16,-0.957716426222737,
-1.69375000000002));
#371459=CARTESIAN_POINT('Ctrl Pts',(0.552937836487023,-0.957716426222737,
-1.65625000000002));
#371460=CARTESIAN_POINT('Ctrl Pts',(0.829406754730535,-0.478858213111369,
-1.61875000000002));
#371461=CARTESIAN_POINT('Ctrl Pts',(1.10587567297405,-3.34922994719732E-16,
-1.58125000000002));
#371462=CARTESIAN_POINT('Ctrl Pts',(0.829406754730536,0.478858213111368,
-1.54375000000002));
#371463=CARTESIAN_POINT('Ctrl Pts',(0.552937836487024,0.957716426222737,
-1.50625000000002));
#371464=CARTESIAN_POINT('Ctrl Pts',(0.,0.957716426222737,-1.46875000000002));
#371465=CARTESIAN_POINT('Ctrl Pts',(-0.552937836487023,0.957716426222737,
-1.43125000000002));
#371466=CARTESIAN_POINT('Ctrl Pts',(-0.829406754730535,0.478858213111368,
-1.39375000000002));
#371467=CARTESIAN_POINT('Ctrl Pts',(-1.10587567297405,-6.38602747653807E-17,
-1.35625000000002));
#371468=CARTESIAN_POINT('Ctrl Pts',(-0.829406754730535,-0.478858213111368,
-1.31875000000002));
#371469=CARTESIAN_POINT('Ctrl Pts',(-0.552937836487024,-0.957716426222737,
-1.28125000000002));
#371470=CARTESIAN_POINT('Ctrl Pts',(-1.17286435586452E-16,-0.957716426222737,
-1.24375000000002));
#371471=CARTESIAN_POINT('Ctrl Pts',(0.552937836487023,-0.957716426222737,
-1.20625000000002));
#371472=CARTESIAN_POINT('Ctrl Pts',(0.829406754730535,-0.478858213111369,
-1.16875000000002));
#371473=CARTESIAN_POINT('Ctrl Pts',(1.10587567297405,-3.34520396076066E-16,
-1.13125000000002));
#371474=CARTESIAN_POINT('Ctrl Pts',(0.829406754730536,0.478858213111368,
-1.09375000000002));
#371475=CARTESIAN_POINT('Ctrl Pts',(0.552937836487024,0.957716426222737,
-1.05625000000002));
#371476=CARTESIAN_POINT('Ctrl Pts',(0.,0.957716426222737,-1.01875000000002));
#371477=CARTESIAN_POINT('Ctrl Pts',(-0.552937836487023,0.957716426222737,
-0.98125000000002));
#371478=CARTESIAN_POINT('Ctrl Pts',(-0.829406754730535,0.478858213111368,
-0.94375000000002));
#371479=CARTESIAN_POINT('Ctrl Pts',(-1.10587567297405,-6.34576761217147E-17,
-0.90625000000002));
#371480=CARTESIAN_POINT('Ctrl Pts',(-0.829406754730535,-0.478858213111368,
-0.86875000000002));
#371481=CARTESIAN_POINT('Ctrl Pts',(-0.552937836487024,-0.957716426222737,
-0.83125000000002));
#371482=CARTESIAN_POINT('Ctrl Pts',(-1.17286435586452E-16,-0.957716426222737,
-0.79375000000002));
#371483=CARTESIAN_POINT('Ctrl Pts',(0.552937836487023,-0.957716426222737,
-0.75625000000002));
#371484=CARTESIAN_POINT('Ctrl Pts',(0.829406754730535,-0.478858213111369,
-0.71875000000002));
#371485=CARTESIAN_POINT('Ctrl Pts',(1.10587567297405,-3.341177974324E-16,
-0.68125000000002));
#371486=CARTESIAN_POINT('Ctrl Pts',(0.829406754730536,0.478858213111368,
-0.64375000000002));
#371487=CARTESIAN_POINT('Ctrl Pts',(0.552937836487024,0.957716426222737,
-0.60625000000002));
#371488=CARTESIAN_POINT('Ctrl Pts',(0.,0.957716426222737,-0.56875000000002));
#371489=CARTESIAN_POINT('Ctrl Pts',(-0.552937836487023,0.957716426222737,
-0.53125000000002));
#371490=CARTESIAN_POINT('Ctrl Pts',(-0.829406754730535,0.478858213111368,
-0.49375000000002));
#371491=CARTESIAN_POINT('Ctrl Pts',(-1.10587567297405,-6.30550774780486E-17,
-0.45625000000002));
#371492=CARTESIAN_POINT('Ctrl Pts',(-0.829406754730535,-0.478858213111368,
-0.41875000000002));
#371493=CARTESIAN_POINT('Ctrl Pts',(-0.552937836487024,-0.957716426222737,
-0.38125000000002));
#371494=CARTESIAN_POINT('Ctrl Pts',(-1.17286435586452E-16,-0.957716426222737,
-0.34375000000002));
#371495=CARTESIAN_POINT('Ctrl Pts',(0.552937836487023,-0.957716426222737,
-0.30625000000002));
#371496=CARTESIAN_POINT('Ctrl Pts',(0.829406754730535,-0.478858213111369,
-0.26875000000002));
#371497=CARTESIAN_POINT('Ctrl Pts',(1.10587567297405,-3.33715198788734E-16,
-0.23125000000002));
#371498=CARTESIAN_POINT('Ctrl Pts',(0.829406754730536,0.478858213111368,
-0.19375000000002));
#371499=CARTESIAN_POINT('Ctrl Pts',(0.552937836487024,0.957716426222737,
-0.15625000000002));
#371500=CARTESIAN_POINT('Ctrl Pts',(0.,0.957716426222737,-0.11875000000002));
#371501=CARTESIAN_POINT('Ctrl Pts',(-0.552937836487023,0.957716426222737,
-0.0812500000000197));
#371502=CARTESIAN_POINT('Ctrl Pts',(-0.829406754730535,0.478858213111368,
-0.0437500000000203));
#371503=CARTESIAN_POINT('Ctrl Pts',(-1.10587567297405,-6.26524788343826E-17,
-0.00625000000002013));
#371504=CARTESIAN_POINT('Ctrl Pts',(-0.829406754730535,-0.478858213111368,
0.0312499999999801));
#371505=CARTESIAN_POINT('Ctrl Pts',(-0.552937836487024,-0.957716426222737,
0.0687499999999803));
#371506=CARTESIAN_POINT('Ctrl Pts',(-1.17286435586452E-16,-0.957716426222737,
0.10624999999998));
#371507=CARTESIAN_POINT('Ctrl Pts',(0.552937836487023,-0.957716426222737,
0.14374999999998));
#371508=CARTESIAN_POINT('Ctrl Pts',(0.829406754730535,-0.478858213111369,
0.18124999999998));
#371509=CARTESIAN_POINT('Ctrl Pts',(1.10587567297405,-3.33312600145068E-16,
0.21874999999998));
#371510=CARTESIAN_POINT('Ctrl Pts',(0.829406754730536,0.478858213111368,
0.25624999999998));
#371511=CARTESIAN_POINT('Ctrl Pts',(0.552937836487024,0.957716426222737,
0.29374999999998));
#371512=CARTESIAN_POINT('Ctrl Pts',(0.,0.957716426222737,0.33124999999998));
#371513=CARTESIAN_POINT('Ctrl Pts',(-0.552937836487023,0.957716426222737,
0.36874999999998));
#371514=CARTESIAN_POINT('Ctrl Pts',(-0.829406754730535,0.478858213111368,
0.40624999999998));
#371515=CARTESIAN_POINT('Ctrl Pts',(-1.10587567297405,-6.22498801907165E-17,
0.44374999999998));
#371516=CARTESIAN_POINT('Ctrl Pts',(-0.829406754730535,-0.478858213111368,
0.48124999999998));
#371517=CARTESIAN_POINT('Ctrl Pts',(-0.552937836487024,-0.957716426222737,
0.51874999999998));
#371518=CARTESIAN_POINT('Ctrl Pts',(-1.17286435586452E-16,-0.957716426222737,
0.556249999999979));
#371519=CARTESIAN_POINT('Ctrl Pts',(0.552937836487023,-0.957716426222737,
0.59374999999998));
#371520=CARTESIAN_POINT('Ctrl Pts',(0.829406754730535,-0.478858213111369,
0.63124999999998));
#371521=CARTESIAN_POINT('Ctrl Pts',(1.10587567297405,-3.32910001501402E-16,
0.66874999999998));
#371522=CARTESIAN_POINT('Ctrl Pts',(0.829406754730536,0.478858213111368,
0.70624999999998));
#371523=CARTESIAN_POINT('Ctrl Pts',(0.552937836487024,0.957716426222737,
0.74374999999998));
#371524=CARTESIAN_POINT('Ctrl Pts',(0.,0.957716426222737,0.78124999999998));
#371525=CARTESIAN_POINT('Ctrl Pts',(-0.552937836487023,0.957716426222737,
0.81874999999998));
#371526=CARTESIAN_POINT('Ctrl Pts',(-0.829406754730535,0.478858213111368,
0.85624999999998));
#371527=CARTESIAN_POINT('Ctrl Pts',(-1.10587567297405,-6.18472815470505E-17,
0.89374999999998));
#371528=CARTESIAN_POINT('Ctrl Pts',(-0.829406754730535,-0.478858213111368,
0.93124999999998));
#371529=CARTESIAN_POINT('Ctrl Pts',(-0.552937836487024,-0.957716426222737,
0.96874999999998));
#371530=CARTESIAN_POINT('Ctrl Pts',(-1.17286435586452E-16,-0.957716426222737,
1.00624999999998));
#371531=CARTESIAN_POINT('Ctrl Pts',(0.552937836487023,-0.957716426222737,
1.04374999999998));
#371532=CARTESIAN_POINT('Ctrl Pts',(0.829406754730535,-0.478858213111369,
1.08124999999998));
#371533=CARTESIAN_POINT('Ctrl Pts',(1.10587567297405,-3.32507402857736E-16,
1.11874999999998));
#371534=CARTESIAN_POINT('Ctrl Pts',(0.829406754730536,0.478858213111368,
1.15624999999998));
#371535=CARTESIAN_POINT('Ctrl Pts',(0.552937836487024,0.957716426222737,
1.19374999999998));
#371536=CARTESIAN_POINT('Ctrl Pts',(0.,0.957716426222737,1.23124999999998));
#371537=CARTESIAN_POINT('Ctrl Pts',(-0.552937836487023,0.957716426222737,
1.26874999999998));
#371538=CARTESIAN_POINT('Ctrl Pts',(-0.829406754730535,0.478858213111368,
1.30624999999998));
#371539=CARTESIAN_POINT('Ctrl Pts',(-1.10587567297405,-6.14446829033844E-17,
1.34374999999998));
#371540=CARTESIAN_POINT('Ctrl Pts',(-0.829406754730535,-0.478858213111368,
1.38124999999998));
#371541=CARTESIAN_POINT('Ctrl Pts',(-0.552937836487024,-0.957716426222737,
1.41874999999998));
#371542=CARTESIAN_POINT('Ctrl Pts',(-1.17286435586452E-16,-0.957716426222737,
1.45624999999998));
#371543=CARTESIAN_POINT('Ctrl Pts',(0.552937836487023,-0.957716426222737,
1.49374999999998));
#371544=CARTESIAN_POINT('Ctrl Pts',(0.829406754730535,-0.478858213111369,
1.53124999999998));
#371545=CARTESIAN_POINT('Ctrl Pts',(1.10587567297405,-3.3210480421407E-16,
1.56874999999998));
#371546=CARTESIAN_POINT('Ctrl Pts',(0.829406754730536,0.478858213111368,
1.60624999999998));
#371547=CARTESIAN_POINT('Ctrl Pts',(0.552937836487024,0.957716426222737,
1.64374999999998));
#371548=CARTESIAN_POINT('Ctrl Pts',(0.,0.957716426222737,1.68124999999998));
#371549=CARTESIAN_POINT('Ctrl Pts',(-0.552937836487023,0.957716426222737,
1.71874999999998));
#371550=CARTESIAN_POINT('Ctrl Pts',(-0.829406754730535,0.478858213111368,
1.75624999999998));
#371551=CARTESIAN_POINT('Ctrl Pts',(-1.10587567297405,-6.10420842597184E-17,
1.79374999999998));
#371552=CARTESIAN_POINT('Ctrl Pts',(-0.829406754730535,-0.478858213111368,
1.83124999999998));
#371553=CARTESIAN_POINT('Ctrl Pts',(-0.552937836487024,-0.957716426222737,
1.86874999999998));
#371554=CARTESIAN_POINT('Ctrl Pts',(-1.17286435586452E-16,-0.957716426222737,
1.90624999999998));
#371555=CARTESIAN_POINT('Ctrl Pts',(0.552937836487023,-0.957716426222737,
1.94374999999998));
#371556=CARTESIAN_POINT('Ctrl Pts',(0.829406754730535,-0.478858213111369,
1.98124999999998));
#371557=CARTESIAN_POINT('Ctrl Pts',(1.10587567297405,-3.31702205570404E-16,
2.01874999999998));
#371558=CARTESIAN_POINT('Ctrl Pts',(0.829406754730536,0.478858213111368,
2.05624999999998));
#371559=CARTESIAN_POINT('Ctrl Pts',(0.552937836487024,0.957716426222737,
2.09374999999998));
#371560=CARTESIAN_POINT('Ctrl Pts',(0.,0.957716426222737,2.13124999999998));
#371561=CARTESIAN_POINT('Ctrl Pts',(-0.552937836487023,0.957716426222737,
2.16874999999998));
#371562=CARTESIAN_POINT('Ctrl Pts',(-0.829406754730535,0.478858213111368,
2.20624999999998));
#371563=CARTESIAN_POINT('Ctrl Pts',(-1.10587567297405,-6.06394856160523E-17,
2.24374999999998));
#371564=CARTESIAN_POINT('Ctrl Pts',(-0.829406754730535,-0.478858213111368,
2.28124999999998));
#371565=CARTESIAN_POINT('Ctrl Pts',(-0.552937836487024,-0.957716426222737,
2.31874999999998));
#371566=CARTESIAN_POINT('Ctrl Pts',(-1.17286435586452E-16,-0.957716426222737,
2.35624999999998));
#371567=CARTESIAN_POINT('Ctrl Pts',(0.552937836487023,-0.957716426222737,
2.39374999999998));
#371568=CARTESIAN_POINT('Ctrl Pts',(0.829406754730535,-0.478858213111369,
2.43124999999998));
#371569=CARTESIAN_POINT('Ctrl Pts',(1.10587567297405,-3.31299606926738E-16,
2.46874999999998));
#371570=CARTESIAN_POINT('Ctrl Pts',(0.829406754730536,0.478858213111368,
2.50624999999998));
#371571=CARTESIAN_POINT('Ctrl Pts',(0.552937836487024,0.957716426222737,
2.54374999999998));
#371572=CARTESIAN_POINT('Ctrl Pts',(0.,0.957716426222737,2.58124999999998));
#371573=CARTESIAN_POINT('Ctrl Pts',(-0.552937836487023,0.957716426222737,
2.61874999999998));
#371574=CARTESIAN_POINT('Ctrl Pts',(-0.829406754730535,0.478858213111368,
2.65624999999998));
#371575=CARTESIAN_POINT('Ctrl Pts',(-1.10587567297405,-6.02368869723863E-17,
2.69374999999998));
#371576=CARTESIAN_POINT('Ctrl Pts',(-0.829406754730535,-0.478858213111368,
2.73124999999998));
#371577=CARTESIAN_POINT('Ctrl Pts',(-0.552937836487024,-0.957716426222737,
2.76874999999998));
#371578=CARTESIAN_POINT('Ctrl Pts',(-1.17286435586452E-16,-0.957716426222737,
2.80624999999998));
#371579=CARTESIAN_POINT('Ctrl Pts',(0.552937836487023,-0.957716426222737,
2.84374999999998));
#371580=CARTESIAN_POINT('Ctrl Pts',(0.829406754730535,-0.478858213111369,
2.88124999999998));
#371581=CARTESIAN_POINT('Ctrl Pts',(1.10587567297405,-3.30897008283072E-16,
2.91874999999998));
#371582=CARTESIAN_POINT('Ctrl Pts',(0.829406754730536,0.478858213111368,
2.95624999999998));
#371583=CARTESIAN_POINT('Ctrl Pts',(0.552937836487024,0.957716426222737,
2.99374999999998));
#371584=CARTESIAN_POINT('Ctrl Pts',(0.,0.957716426222737,3.03124999999998));
#371585=CARTESIAN_POINT('Ctrl Pts',(-0.552937836487023,0.957716426222737,
3.06874999999998));
#371586=CARTESIAN_POINT('Ctrl Pts',(-0.829406754730535,0.478858213111368,
3.10624999999998));
#371587=CARTESIAN_POINT('Ctrl Pts',(-1.10587567297405,-5.98342883287202E-17,
3.14374999999998));
#371588=CARTESIAN_POINT('Ctrl Pts',(-0.829406754730535,-0.478858213111368,
3.18124999999998));
#371589=CARTESIAN_POINT('Ctrl Pts',(-0.552937836487024,-0.957716426222737,
3.21874999999998));
#371590=CARTESIAN_POINT('Ctrl Pts',(-1.17286435586452E-16,-0.957716426222737,
3.25624999999998));
#371591=CARTESIAN_POINT('Ctrl Pts',(0.552937836487023,-0.957716426222737,
3.29374999999998));
#371592=CARTESIAN_POINT('Ctrl Pts',(0.829406754730535,-0.478858213111369,
3.33124999999998));
#371593=CARTESIAN_POINT('Ctrl Pts',(1.10587567297405,-3.30494409639406E-16,
3.36874999999998));
#371594=CARTESIAN_POINT('Ctrl Pts',(0.829406754730536,0.478858213111368,
3.40624999999998));
#371595=CARTESIAN_POINT('Ctrl Pts',(0.552937836487024,0.957716426222737,
3.44374999999998));
#371596=CARTESIAN_POINT('Ctrl Pts',(0.,0.957716426222737,3.48124999999998));
#371597=CARTESIAN_POINT('Ctrl Pts',(-0.552937836487023,0.957716426222737,
3.51874999999998));
#371598=CARTESIAN_POINT('Ctrl Pts',(-0.829406754730535,0.478858213111368,
3.55624999999998));
#371599=CARTESIAN_POINT('Ctrl Pts',(-1.10587567297405,-5.94316896850542E-17,
3.59374999999998));
#371600=CARTESIAN_POINT('Ctrl Pts',(-0.829406754730535,-0.478858213111368,
3.63124999999998));
#371601=CARTESIAN_POINT('Ctrl Pts',(-0.552937836487024,-0.957716426222737,
3.66874999999998));
#371602=CARTESIAN_POINT('Ctrl Pts',(-1.17286435586452E-16,-0.957716426222737,
3.70624999999998));
#371603=CARTESIAN_POINT('Ctrl Pts',(0.552937836487023,-0.957716426222737,
3.74374999999998));
#371604=CARTESIAN_POINT('Ctrl Pts',(0.829406754730535,-0.478858213111369,
3.78124999999998));
#371605=CARTESIAN_POINT('Ctrl Pts',(1.00369205912859,-0.176987210881325,
3.80488990482708));
#371606=CARTESIAN_POINT('Ctrl Pts',(0.94316952501371,0.16628890564997,3.83177229718761));
#459207=UNCERTAINTY_MEASURE_WITH_UNIT(LENGTH_MEASURE(0.01),#459243,
'DISTANCE_ACCURACY_VALUE',
'Maximum model space distance between geometric entities at asserted c
onnectivities');
#459216=UNCERTAINTY_MEASURE_WITH_UNIT(LENGTH_MEASURE(0.01),#459243,
'DISTANCE_ACCURACY_VALUE',
'Maximum model space distance between geometric entities at asserted c
onnectivities');
#459233=(
GEOMETRIC_REPRESENTATION_CONTEXT(3)
GLOBAL_UNCERTAINTY_ASSIGNED_CONTEXT((#459207))
GLOBAL_UNIT_ASSIGNED_CONTEXT((#459243,#459245,#459246))
REPRESENTATION_CONTEXT('','3D')
);
#459242=(
GEOMETRIC_REPRESENTATION_CONTEXT(3)
GLOBAL_UNCERTAINTY_ASSIGNED_CONTEXT((#459216))
GLOBAL_UNIT_ASSIGNED_CONTEXT((#459243,#459245,#459246))
REPRESENTATION_CONTEXT('','3D')
);
#459243=(
LENGTH_UNIT()
NAMED_UNIT(*)
SI_UNIT(.MILLI.,.METRE.)
);
#459245=(
NAMED_UNIT(*)
PLANE_ANGLE_UNIT()
SI_UNIT($,.RADIAN.)
);
#459246=(
NAMED_UNIT(*)
SI_UNIT($,.STERADIAN.)
SOLID_ANGLE_UNIT()
);
#459263=SHAPE_DEFINITION_REPRESENTATION(#459290,#459344);
#459290=PRODUCT_DEFINITION_SHAPE('',$,#459370);
#459344=SHAPE_REPRESENTATION('',(#99318),#459233);
#459353=PRODUCT_DEFINITION_CONTEXT('part definition',#459430,'design');
#459370=PRODUCT_DEFINITION('Housing Fastener','Housing Fastener',#459395,
#459353);
#459395=PRODUCT_DEFINITION_FORMATION('',$,#459448);
#459430=APPLICATION_CONTEXT(
'Core Data for Automotive Mechanical Design Process');
#459431=PRODUCT_CONTEXT('part definition',#459430,'mechanical');
#459448=PRODUCT('Housing Fastener','Housing Fastener',$,(#459431));
#459527=COLOUR_RGB('Black',0.12,0.14,0.17);
#459528=FILL_AREA_STYLE_COLOUR('',#459527);
#459529=FILL_AREA_STYLE('',(#459528));
#459530=SURFACE_STYLE_FILL_AREA(#459529);
#459531=SURFACE_SIDE_STYLE('',(#459530));
#459532=SURFACE_STYLE_USAGE(.BOTH.,#459531);
#459533=PRESENTATION_STYLE_ASSIGNMENT((#459532));
ENDSEC;
END-ISO-10303-21;
